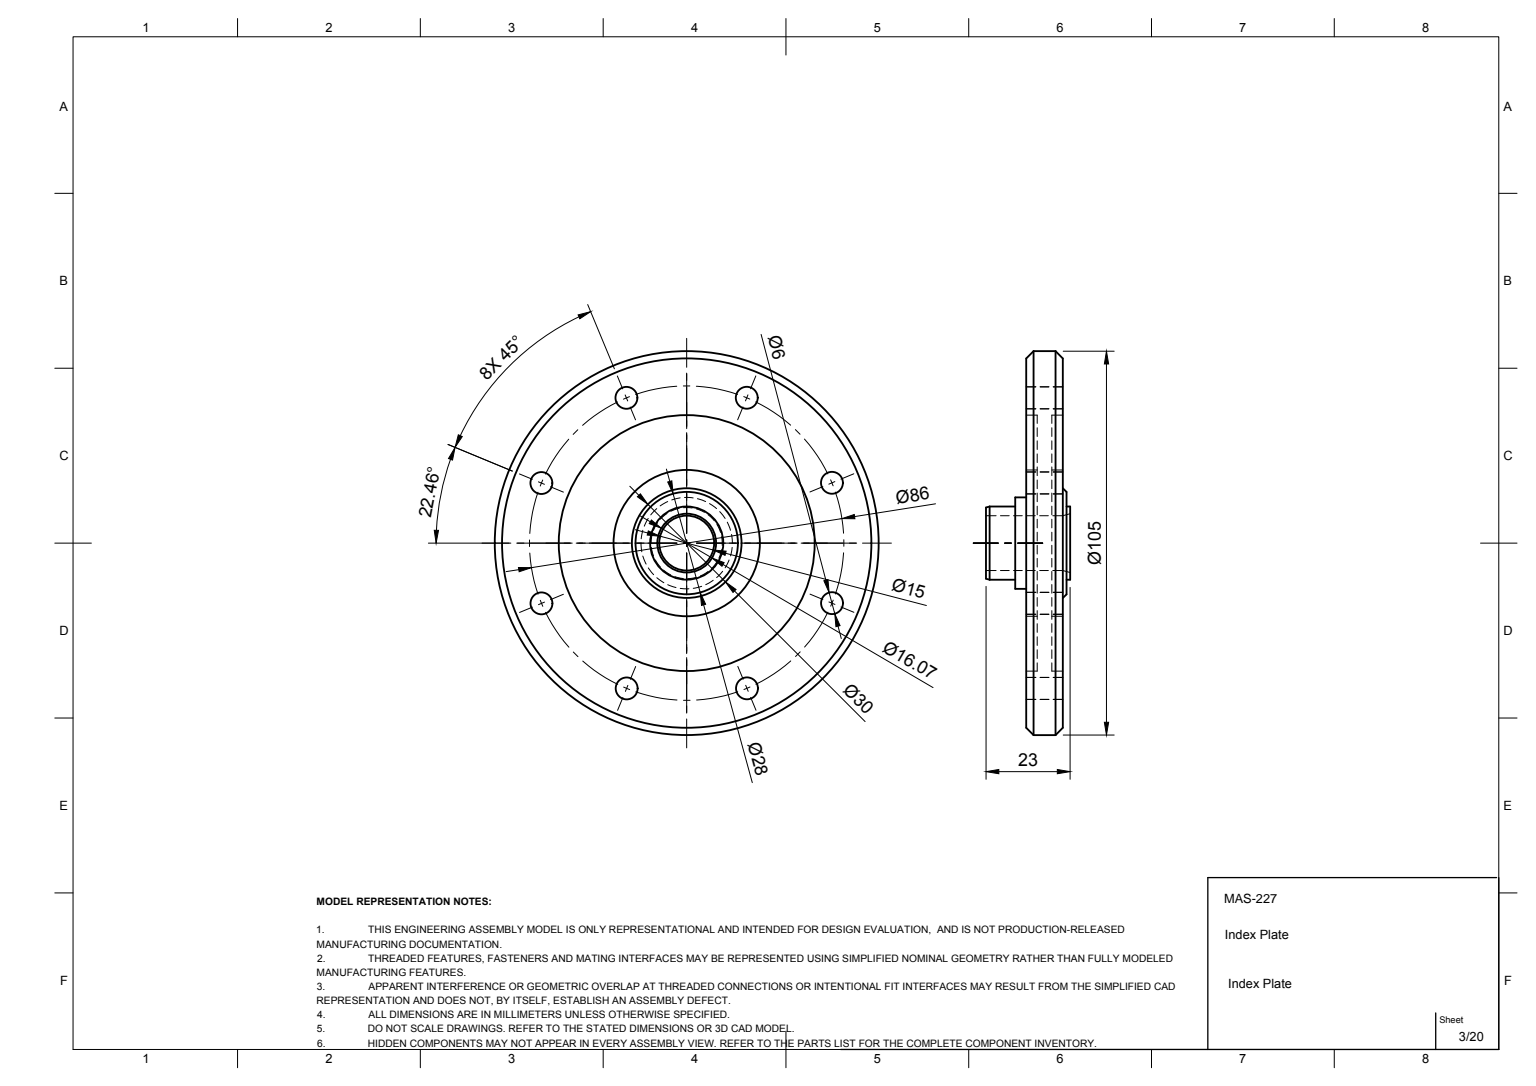
ISO-10303-21;
HEADER;
FILE_DESCRIPTION (('STEP AP214'),
    '1' );
FILE_NAME ( 'Index Plate.step', '2026-10-06T08:24:41', ( '' ), ( '' ), 'STEP AP214', 'Unspecified', '' );
FILE_SCHEMA (( 'AUTOMOTIVE_DESIGN' ));
ENDSEC;
DATA;
#10=DIRECTION ( 'NONE',  ( 0.000000000000000000, 0.000000000000000000, -1.000000000000000000 ) ) ;
#33=EDGE_CURVE ( 'NONE', #1582, #19320, #13242, .T. ) ;
#44=DIRECTION ( 'NONE',  ( -0.000000000000000000, -1.000000000000000000, -0.000000000000000000 ) ) ;
#78=VECTOR ( 'NONE', #27167, 39.37007874015748854 ) ;
#114=EDGE_CURVE ( 'NONE', #14474, #3555, #20012, .T. ) ;
#152=VERTEX_POINT ( 'NONE', #7235 ) ;
#164=CIRCLE ( 'NONE', #26696, 1.988188976448617584 ) ;
#176=ADVANCED_FACE ( 'NONE', ( #13590 ), #15218, .F. ) ;
#177=DIRECTION ( 'NONE',  ( 0.000000000000000000, 0.000000000000000000, 1.000000000000000000 ) ) ;
#193=CIRCLE ( 'NONE', #14146, 0.1181102362204720091 ) ;
#200=DIRECTION ( 'NONE',  ( 0.000000000000000000, -1.000000000000000000, 0.000000000000000000 ) ) ;
#201=DIRECTION ( 'NONE',  ( -0.000000000000000000, -1.000000000000000000, -0.000000000000000000 ) ) ;
#202=DIRECTION ( 'NONE',  ( 0.000000000000000000, 0.000000000000000000, 1.000000000000000000 ) ) ;
#247=VERTEX_POINT ( 'NONE', #23212 ) ;
#249=ORIENTED_EDGE ( 'NONE', *, *, #1427, .F. ) ;
#264=DIRECTION ( 'NONE',  ( -0.000000000000000000, -1.000000000000000000, -0.000000000000000000 ) ) ;
#291=ORIENTED_EDGE ( 'NONE', *, *, #20836, .F. ) ;
#298=EDGE_CURVE ( 'NONE', #7459, #10848, #1546, .T. ) ;
#311=ORIENTED_EDGE ( 'NONE', *, *, #16319, .F. ) ;
#320=ORIENTED_EDGE ( 'NONE', *, *, #13672, .F. ) ;
#353=DIRECTION ( 'NONE',  ( -0.000000000000000000, 1.000000000000000000, -0.000000000000000000 ) ) ;
#372=VERTEX_POINT ( 'NONE', #12604 ) ;
#378=CARTESIAN_POINT ( 'NONE',  ( 0.000000000000000000, 0.07874015746264864668, 0.000000000000000000 ) ) ;
#384=SURFACE_SIDE_STYLE ('',( #2200 ) ) ;
#403=CARTESIAN_POINT ( 'NONE',  ( 0.000000000000000000, 0.3543307086614173040, 0.000000000000000000 ) ) ;
#406=ORIENTED_EDGE ( 'NONE', *, *, #12519, .T. ) ;
#415=CARTESIAN_POINT ( 'NONE',  ( 0.000000000000000000, 0.1574803148899641958, 0.000000000000000000 ) ) ;
#436=CARTESIAN_POINT ( 'NONE',  ( 0.000000000000000000, 0.4724409448818898127, 0.000000000000000000 ) ) ;
#464=ADVANCED_FACE ( 'NONE', ( #6671 ), #22286, .T. ) ;
#482=CARTESIAN_POINT ( 'NONE',  ( 1.197070535079588716, 0.4724409448818898127, -1.315180771300060503 ) ) ;
#493=EDGE_LOOP ( 'NONE', ( #11745, #14981, #2623, #22261 ) ) ;
#508=AXIS2_PLACEMENT_3D ( 'NONE', #15619, #21831, #3001 ) ;
#514=CARTESIAN_POINT ( 'NONE',  ( 7.232166136913317628E-17, 0.07874015746264864668, -0.5905511811200284678 ) ) ;
#529=AXIS2_PLACEMENT_3D ( 'NONE', #1743, #21245, #23088 ) ;
#629=ORIENTED_EDGE ( 'NONE', *, *, #18848, .T. ) ;
#694=DIRECTION ( 'NONE',  ( -0.000000000000000000, -1.000000000000000000, -0.000000000000000000 ) ) ;
#697=ORIENTED_EDGE ( 'NONE', *, *, #23351, .F. ) ;
#706=DIRECTION ( 'NONE',  ( -0.000000000000000000, -1.000000000000000000, -0.000000000000000000 ) ) ;
#709=EDGE_CURVE ( 'NONE', #4045, #152, #22753, .T. ) ;
#726=DIRECTION ( 'NONE',  ( 0.000000000000000000, 0.000000000000000000, -1.000000000000000000 ) ) ;
#755=DIRECTION ( 'NONE',  ( -0.000000000000000000, -1.000000000000000000, -0.000000000000000000 ) ) ;
#759=PLANE ( 'NONE',  #24631 ) ;
#789=ORIENTED_EDGE ( 'NONE', *, *, #20752, .F. ) ;
#799=ORIENTED_EDGE ( 'NONE', *, *, #16948, .T. ) ;
#837=CYLINDRICAL_SURFACE ( 'NONE', #12003, 0.1181102362204718703 ) ;
#847=CARTESIAN_POINT ( 'NONE',  ( -2.073220866141732523E-16, 0.4724409448818898127, 1.692913385826771533 ) ) ;
#857=UNCERTAINTY_MEASURE_WITH_UNIT (LENGTH_MEASURE( 1.000000000000000082E-05 ), #18780, 'distance_accuracy_value', 'NONE') ;
#865=CIRCLE ( 'NONE', #10326, 0.1181102362204720091 ) ;
#870=ORIENTED_EDGE ( 'NONE', *, *, #1826, .T. ) ;
#892=DIRECTION ( 'NONE',  ( 0.000000000000000000, -1.000000000000000000, 0.000000000000000000 ) ) ;
#894=CIRCLE ( 'NONE', #26579, 0.1181102362204718703 ) ;
#911=EDGE_LOOP ( 'NONE', ( #11469, #21986 ) ) ;
#938=EDGE_LOOP ( 'NONE', ( #21430, #4636, #799, #17993 ) ) ;
#965=DIRECTION ( 'NONE',  ( 0.000000000000000000, 0.000000000000000000, -1.000000000000000000 ) ) ;
#978=AXIS2_PLACEMENT_3D ( 'NONE', #24637, #18270, #11515 ) ;
#1000=DIRECTION ( 'NONE',  ( 0.000000000000000000, -1.000000000000000000, 0.000000000000000000 ) ) ;
#1003=CARTESIAN_POINT ( 'NONE',  ( 0.000000000000000000, 0.4724409448818898127, 0.000000000000000000 ) ) ;
#1012=CARTESIAN_POINT ( 'NONE',  ( 1.197070535079588716, 0.4724409448818898127, 1.197070535079588716 ) ) ;
#1027=AXIS2_PLACEMENT_3D ( 'NONE', #3554, #3412, #20244 ) ;
#1082=CIRCLE ( 'NONE', #11898, 0.1181102362204720091 ) ;
#1086=VERTEX_POINT ( 'NONE', #20162 ) ;
#1089=ORIENTED_EDGE ( 'NONE', *, *, #4333, .F. ) ;
#1107=CARTESIAN_POINT ( 'NONE',  ( -2.073220866141732523E-16, 0.07874015748031495954, 1.574803149606299524 ) ) ;
#1178=CARTESIAN_POINT ( 'NONE',  ( 0.000000000000000000, 0.03937007874015751446, 0.5511811023975373702 ) ) ;
#1184=ORIENTED_EDGE ( 'NONE', *, *, #12547, .T. ) ;
#1222=CARTESIAN_POINT ( 'NONE',  ( 0.000000000000000000, 0.4724409448818898127, 1.377952755905512472 ) ) ;
#1244=FACE_OUTER_BOUND ( 'NONE', #1397, .T. ) ;
#1249=EDGE_CURVE ( 'NONE', #21158, #7057, #2465, .T. ) ;
#1250=EDGE_LOOP ( 'NONE', ( #8180, #21295, #4670, #1522 ) ) ;
#1298=DIRECTION ( 'NONE',  ( 0.000000000000000000, 0.000000000000000000, -1.000000000000000000 ) ) ;
#1310=AXIS2_PLACEMENT_3D ( 'NONE', #22025, #2927, #13675 ) ;
#1323=DIRECTION ( 'NONE',  ( 0.000000000000000000, -1.000000000000000000, 0.000000000000000000 ) ) ;
#1331=LINE ( 'NONE', #14195, #11270 ) ;
#1353=CIRCLE ( 'NONE', #24413, 0.1181102362204718703 ) ;
#1389=AXIS2_PLACEMENT_3D ( 'NONE', #415, #8594, #17214 ) ;
#1396=ADVANCED_FACE ( 'NONE', ( #19306 ), #27299, .F. ) ;
#1397=EDGE_LOOP ( 'NONE', ( #19459, #25159, #1953, #13540 ) ) ;
#1405=DIRECTION ( 'NONE',  ( 0.000000000000000000, 0.000000000000000000, -1.000000000000000000 ) ) ;
#1406=FACE_OUTER_BOUND ( 'NONE', #22178, .T. ) ;
#1427=EDGE_CURVE ( 'NONE', #13858, #1638, #10407, .T. ) ;
#1432=ORIENTED_EDGE ( 'NONE', *, *, #27506, .F. ) ;
#1439=FACE_OUTER_BOUND ( 'NONE', #16521, .T. ) ;
#1469=DIRECTION ( 'NONE',  ( 0.000000000000000000, 0.000000000000000000, 1.000000000000000000 ) ) ;
#1498=VERTEX_POINT ( 'NONE', #23836 ) ;
#1522=ORIENTED_EDGE ( 'NONE', *, *, #5885, .F. ) ;
#1546=CIRCLE ( 'NONE', #3787, 2.066929133858267598 ) ;
#1552=CYLINDRICAL_SURFACE ( 'NONE', #2874, 0.4921259842519685179 ) ;
#1553=CIRCLE ( 'NONE', #15987, 0.1181102362204718703 ) ;
#1582=VERTEX_POINT ( 'NONE', #514 ) ;
#1595=EDGE_LOOP ( 'NONE', ( #26419, #5301, #7926, #27061 ) ) ;
#1610=CARTESIAN_POINT ( 'NONE',  ( 1.197070535079588716, 0.4724409448818898127, -1.078960298859116707 ) ) ;
#1616=CIRCLE ( 'NONE', #19678, 0.5905511811200284678 ) ;
#1635=VECTOR ( 'NONE', #4381, 39.37007874015748143 ) ;
#1636=ORIENTED_EDGE ( 'NONE', *, *, #27592, .T. ) ;
#1638=VERTEX_POINT ( 'NONE', #14061 ) ;
#1662=ORIENTED_EDGE ( 'NONE', *, *, #10822, .F. ) ;
#1672=FACE_BOUND ( 'NONE', #15271, .T. ) ;
#1726=ADVANCED_FACE ( 'NONE', ( #26317 ), #15603, .F. ) ;
#1743=CARTESIAN_POINT ( 'NONE',  ( 1.197070535079588716, 0.07874015748031491790, 1.197070535079588716 ) ) ;
#1776=EDGE_LOOP ( 'NONE', ( #5191, #3229 ) ) ;
#1790=ORIENTED_EDGE ( 'NONE', *, *, #19478, .T. ) ;
#1813=FACE_BOUND ( 'NONE', #23770, .T. ) ;
#1820=CYLINDRICAL_SURFACE ( 'NONE', #15991, 0.1181102362204718703 ) ;
#1824=ORIENTED_EDGE ( 'NONE', *, *, #3257, .F. ) ;
#1826=EDGE_CURVE ( 'NONE', #17190, #19458, #11615, .T. ) ;
#1845=DIRECTION ( 'NONE',  ( 0.000000000000000000, -1.000000000000000000, 0.000000000000000000 ) ) ;
#1864=CIRCLE ( 'NONE', #3209, 0.1181102362204718703 ) ;
#1930=AXIS2_PLACEMENT_3D ( 'NONE', #8276, #16896, #4038 ) ;
#1938=EDGE_LOOP ( 'NONE', ( #18405, #23530, #16825, #17076 ) ) ;
#1939=AXIS2_PLACEMENT_3D ( 'NONE', #16280, #5401, #14020 ) ;
#1953=ORIENTED_EDGE ( 'NONE', *, *, #18523, .F. ) ;
#1991=ORIENTED_EDGE ( 'NONE', *, *, #20752, .T. ) ;
#2060=VECTOR ( 'NONE', #15684, 39.37007874015748143 ) ;
#2102=CARTESIAN_POINT ( 'NONE',  ( 0.000000000000000000, 0.9055118110236221041, 0.000000000000000000 ) ) ;
#2122=ORIENTED_EDGE ( 'NONE', *, *, #5680, .F. ) ;
#2124=AXIS2_PLACEMENT_3D ( 'NONE', #13217, #12672, #11106 ) ;
#2135=ORIENTED_EDGE ( 'NONE', *, *, #21289, .T. ) ;
#2145=( GEOMETRIC_REPRESENTATION_CONTEXT ( 3 ) GLOBAL_UNCERTAINTY_ASSIGNED_CONTEXT ( ( #24851 ) ) GLOBAL_UNIT_ASSIGNED_CONTEXT ( ( #26069, #23822, #10819 ) ) REPRESENTATION_CONTEXT ( 'NONE', 'WORKASPACE' ) ) ;
#2170=CARTESIAN_POINT ( 'NONE',  ( 0.000000000000000000, 0.07874015748662489822, 0.000000000000000000 ) ) ;
#2181=EDGE_LOOP ( 'NONE', ( #2379, #22153 ) ) ;
#2186=LINE ( 'NONE', #14929, #19182 ) ;
#2194=LINE ( 'NONE', #8827, #18525 ) ;
#2200=SURFACE_STYLE_FILL_AREA ( #4325 ) ;
#2225=VERTEX_POINT ( 'NONE', #20456 ) ;
#2314=FACE_OUTER_BOUND ( 'NONE', #19001, .T. ) ;
#2328=( LENGTH_UNIT ( ) NAMED_UNIT ( * ) SI_UNIT ( $, .METRE. ) ) ;
#2332=CYLINDRICAL_SURFACE ( 'NONE', #25371, 0.1181102362204718703 ) ;
#2379=ORIENTED_EDGE ( 'NONE', *, *, #15595, .T. ) ;
#2409=AXIS2_PLACEMENT_3D ( 'NONE', #403, #13231, #17610 ) ;
#2460=DIRECTION ( 'NONE',  ( 0.000000000000000000, 0.000000000000000000, -1.000000000000000000 ) ) ;
#2465=CIRCLE ( 'NONE', #2913, 1.988188976307287970 ) ;
#2480=ORIENTED_EDGE ( 'NONE', *, *, #12460, .F. ) ;
#2514=CIRCLE ( 'NONE', #22359, 0.1181102362204718703 ) ;
#2527=DIRECTION ( 'NONE',  ( 0.000000000000000000, 0.000000000000000000, -1.000000000000000000 ) ) ;
#2543=CARTESIAN_POINT ( 'NONE',  ( 1.692913385826771533, 0.4724409448818898127, 0.1181102362204723144 ) ) ;
#2550=EDGE_LOOP ( 'NONE', ( #23716, #23135, #18608, #25264 ) ) ;
#2576=APPLICATION_CONTEXT ( 'automotive_design' ) ;
#2623=ORIENTED_EDGE ( 'NONE', *, *, #25477, .T. ) ;
#2674=ADVANCED_FACE ( 'NONE', ( #8431 ), #10402, .T. ) ;
#2689=ORIENTED_EDGE ( 'NONE', *, *, #22485, .T. ) ;
#2707=MANIFOLD_SOLID_BREP ( 'Index Plate', #6943 ) ;
#2718=ORIENTED_EDGE ( 'NONE', *, *, #10592, .T. ) ;
#2741=CIRCLE ( 'NONE', #978, 0.3831516066089791228 ) ;
#2769=FACE_OUTER_BOUND ( 'NONE', #11806, .T. ) ;
#2772=CONICAL_SURFACE ( 'NONE', #11805, 1.988188976307287970, 0.7853981642948970610 ) ;
#2776=DIRECTION ( 'NONE',  ( -0.000000000000000000, 1.000000000000000000, -0.000000000000000000 ) ) ;
#2782=LINE ( 'NONE', #11011, #8118 ) ;
#2784=EDGE_CURVE ( 'NONE', #13707, #10268, #25934, .T. ) ;
#2794=CIRCLE ( 'NONE', #3231, 0.7874015748031496509 ) ;
#2796=CARTESIAN_POINT ( 'NONE',  ( 0.000000000000000000, 0.1968503937007874127, -0.3937007874015748254 ) ) ;
#2812=EDGE_CURVE ( 'NONE', #2225, #7703, #23380, .T. ) ;
#2835=CARTESIAN_POINT ( 'NONE',  ( 0.000000000000000000, 0.07874015746264864668, 0.5905511811200284678 ) ) ;
#2845=LINE ( 'NONE', #11483, #16951 ) ;
#2851=DIRECTION ( 'NONE',  ( 0.000000000000000000, 0.000000000000000000, -1.000000000000000000 ) ) ;
#2874=AXIS2_PLACEMENT_3D ( 'NONE', #10156, #27408, #8066 ) ;
#2875=ORIENTED_EDGE ( 'NONE', *, *, #4475, .T. ) ;
#2878=AXIS2_PLACEMENT_3D ( 'NONE', #378, #3646, #18474 ) ;
#2898=ORIENTED_EDGE ( 'NONE', *, *, #24019, .F. ) ;
#2913=AXIS2_PLACEMENT_3D ( 'NONE', #14096, #26953, #965 ) ;
#2927=DIRECTION ( 'NONE',  ( -0.000000000000000000, -1.000000000000000000, -0.000000000000000000 ) ) ;
#2933=DIMENSIONAL_EXPONENTS ( 1.000000000000000000, 0.000000000000000000, 0.000000000000000000, 0.000000000000000000, 0.000000000000000000, 0.000000000000000000, 0.000000000000000000 ) ;
#2961=EDGE_LOOP ( 'NONE', ( #5163, #7139, #19666, #17295 ) ) ;
#2970=EDGE_LOOP ( 'NONE', ( #22132, #13262 ) ) ;
#2973=EDGE_CURVE ( 'NONE', #18986, #1498, #26337, .T. ) ;
#3000=DIRECTION ( 'NONE',  ( -0.000000000000000000, -1.000000000000000000, -0.000000000000000000 ) ) ;
#3001=DIRECTION ( 'NONE',  ( 0.000000000000000000, 0.000000000000000000, -1.000000000000000000 ) ) ;
#3013=STYLED_ITEM ( 'NONE', ( #6589 ), #2707 ) ;
#3036=AXIS2_PLACEMENT_3D ( 'NONE', #19500, #25728, #6375 ) ;
#3043=DIRECTION ( 'NONE',  ( -0.000000000000000000, -1.000000000000000000, -0.000000000000000000 ) ) ;
#3055=AXIS2_PLACEMENT_3D ( 'NONE', #14460, #3688, #12316 ) ;
#3068=EDGE_LOOP ( 'NONE', ( #12674, #2875, #25773, #20146 ) ) ;
#3069=ADVANCED_FACE ( 'NONE', ( #6279 ), #14838, .F. ) ;
#3070=ORIENTED_EDGE ( 'NONE', *, *, #9051, .T. ) ;
#3095=LENGTH_MEASURE_WITH_UNIT ( LENGTH_MEASURE( 0.02539999999999999897 ), #22747 ) ;
#3120=EDGE_CURVE ( 'NONE', #7099, #13627, #22918, .T. ) ;
#3122=AXIS2_PLACEMENT_3D ( 'NONE', #20332, #24693, #13985 ) ;
#3168=DIRECTION ( 'NONE',  ( 0.000000000000000000, -1.000000000000000000, 0.000000000000000000 ) ) ;
#3201=VERTEX_POINT ( 'NONE', #18103 ) ;
#3209=AXIS2_PLACEMENT_3D ( 'NONE', #3734, #14648, #3882 ) ;
#3216=CARTESIAN_POINT ( 'NONE',  ( 0.000000000000000000, 0.5905511811023621549, 0.000000000000000000 ) ) ;
#3223=CARTESIAN_POINT ( 'NONE',  ( -1.197070535079588716, 0.4724409448818898127, -1.078960298859116707 ) ) ;
#3224=FACE_OUTER_BOUND ( 'NONE', #18819, .T. ) ;
#3229=ORIENTED_EDGE ( 'NONE', *, *, #19328, .T. ) ;
#3231=AXIS2_PLACEMENT_3D ( 'NONE', #10033, #1845, #10310 ) ;
#3244=ADVANCED_FACE ( 'NONE', ( #18257 ), #7258, .F. ) ;
#3245=DIRECTION ( 'NONE',  ( 0.000000000000000000, 0.000000000000000000, -1.000000000000000000 ) ) ;
#3257=EDGE_CURVE ( 'NONE', #372, #13858, #19762, .T. ) ;
#3379=VECTOR ( 'NONE', #4006, 39.37007874015748854 ) ;
#3403=DIRECTION ( 'NONE',  ( -0.000000000000000000, -1.000000000000000000, -0.000000000000000000 ) ) ;
#3412=DIRECTION ( 'NONE',  ( -0.000000000000000000, 1.000000000000000000, -0.000000000000000000 ) ) ;
#3415=EDGE_LOOP ( 'NONE', ( #27420, #16968 ) ) ;
#3459=EDGE_LOOP ( 'NONE', ( #14828, #18126 ) ) ;
#3471=CARTESIAN_POINT ( 'NONE',  ( 1.446433227339386678E-17, 0.4724409448818898127, -1.574803149606299524 ) ) ;
#3477=ORIENTED_EDGE ( 'NONE', *, *, #8160, .T. ) ;
#3478=DIRECTION ( 'NONE',  ( 0.000000000000000000, -1.000000000000000000, 0.000000000000000000 ) ) ;
#3479=DIRECTION ( 'NONE',  ( -0.000000000000000000, -1.000000000000000000, -0.000000000000000000 ) ) ;
#3480=DIRECTION ( 'NONE',  ( 0.000000000000000000, -0.9659258263664941557, -0.2588190448135637145 ) ) ;
#3494=EDGE_CURVE ( 'NONE', #23576, #24515, #4893, .T. ) ;
#3513=DIRECTION ( 'NONE',  ( -0.000000000000000000, -1.000000000000000000, -0.000000000000000000 ) ) ;
#3525=DIRECTION ( 'NONE',  ( -0.000000000000000000, -1.000000000000000000, -0.000000000000000000 ) ) ;
#3530=AXIS2_PLACEMENT_3D ( 'NONE', #9173, #7487, #22603 ) ;
#3544=LINE ( 'NONE', #5262, #78 ) ;
#3551=VECTOR ( 'NONE', #16165, 39.37007874015748143 ) ;
#3554=CARTESIAN_POINT ( 'NONE',  ( 0.000000000000000000, 0.4724409448818896462, 0.000000000000000000 ) ) ;
#3555=VERTEX_POINT ( 'NONE', #1610 ) ;
#3606=ADVANCED_BREP_SHAPE_REPRESENTATION ( 'Index Plate', ( #2707, #11588 ), #8455 ) ;
#3618=CIRCLE ( 'NONE', #21691, 0.3937007874015748254 ) ;
#3638=ORIENTED_EDGE ( 'NONE', *, *, #20353, .F. ) ;
#3646=DIRECTION ( 'NONE',  ( 0.000000000000000000, -1.000000000000000000, 0.000000000000000000 ) ) ;
#3665=DIRECTION ( 'NONE',  ( 0.000000000000000000, 0.000000000000000000, 1.000000000000000000 ) ) ;
#3672=CARTESIAN_POINT ( 'NONE',  ( -1.692913385826771533, 0.07874015748031491790, 0.1181102362204718981 ) ) ;
#3680=CYLINDRICAL_SURFACE ( 'NONE', #9596, 0.1181102362204718703 ) ;
#3685=EDGE_CURVE ( 'NONE', #16564, #8713, #6703, .T. ) ;
#3688=DIRECTION ( 'NONE',  ( 0.000000000000000000, -1.000000000000000000, 0.000000000000000000 ) ) ;
#3695=CIRCLE ( 'NONE', #2409, 0.7874015748031496509 ) ;
#3716=FACE_OUTER_BOUND ( 'NONE', #16941, .T. ) ;
#3734=CARTESIAN_POINT ( 'NONE',  ( -1.197070535079588716, 0.07874015748031491790, -1.197070535079588716 ) ) ;
#3736=ORIENTED_EDGE ( 'NONE', *, *, #298, .F. ) ;
#3749=CARTESIAN_POINT ( 'NONE',  ( 0.000000000000000000, 0.5905511811023621549, 0.000000000000000000 ) ) ;
#3762=CARTESIAN_POINT ( 'NONE',  ( 0.000000000000000000, 0.3543307086614172485, 1.377952755905512472 ) ) ;
#3787=AXIS2_PLACEMENT_3D ( 'NONE', #6123, #7950, #14758 ) ;
#3794=ORIENTED_EDGE ( 'NONE', *, *, #11136, .F. ) ;
#3815=CARTESIAN_POINT ( 'NONE',  ( 4.756848988674917118E-17, 0.9055118110236221041, 0.3831516066089791228 ) ) ;
#3846=VECTOR ( 'NONE', #3403, 39.37007874015748143 ) ;
#3856=CARTESIAN_POINT ( 'NONE',  ( 0.000000000000000000, 0.07874015748662489822, 0.000000000000000000 ) ) ;
#3866=DIRECTION ( 'NONE',  ( 0.000000000000000000, -1.000000000000000000, 0.000000000000000000 ) ) ;
#3882=DIRECTION ( 'NONE',  ( 0.000000000000000000, 0.000000000000000000, -1.000000000000000000 ) ) ;
#3899=CARTESIAN_POINT ( 'NONE',  ( 0.000000000000000000, 0.07874015748031491790, -1.692913385826771533 ) ) ;
#3906=FACE_OUTER_BOUND ( 'NONE', #14752, .T. ) ;
#3934=VERTEX_POINT ( 'NONE', #19157 ) ;
#3937=DIRECTION ( 'NONE',  ( -0.000000000000000000, 1.000000000000000000, -0.000000000000000000 ) ) ;
#3946=ORIENTED_EDGE ( 'NONE', *, *, #16858, .F. ) ;
#3956=DIRECTION ( 'NONE',  ( 0.000000000000000000, 0.000000000000000000, -1.000000000000000000 ) ) ;
#3960=EDGE_LOOP ( 'NONE', ( #697, #25923 ) ) ;
#3981=ORIENTED_EDGE ( 'NONE', *, *, #2973, .F. ) ;
#4006=DIRECTION ( 'NONE',  ( 0.000000000000000000, -0.9659258263664933786, -0.2588190448135661570 ) ) ;
#4038=DIRECTION ( 'NONE',  ( 0.000000000000000000, 0.000000000000000000, -1.000000000000000000 ) ) ;
#4045=VERTEX_POINT ( 'NONE', #18047 ) ;
#4048=DIRECTION ( 'NONE',  ( 0.000000000000000000, 1.000000000000000000, 0.000000000000000000 ) ) ;
#4055=FACE_OUTER_BOUND ( 'NONE', #10449, .T. ) ;
#4060=ADVANCED_FACE ( 'NONE', ( #1244 ), #7157, .T. ) ;
#4079=CARTESIAN_POINT ( 'NONE',  ( 0.000000000000000000, 0.3543307086614172485, 0.000000000000000000 ) ) ;
#4125=FACE_OUTER_BOUND ( 'NONE', #4418, .T. ) ;
#4141=ORIENTED_EDGE ( 'NONE', *, *, #22416, .F. ) ;
#4161=CIRCLE ( 'NONE', #7316, 0.3937007874015748254 ) ;
#4228=FACE_OUTER_BOUND ( 'NONE', #1938, .T. ) ;
#4269=AXIS2_PLACEMENT_3D ( 'NONE', #3856, #1323, #16998 ) ;
#4325=FILL_AREA_STYLE ('',( #23421 ) ) ;
#4333=EDGE_CURVE ( 'NONE', #27329, #8591, #12247, .T. ) ;
#4366=CIRCLE ( 'NONE', #14290, 0.3937007874015748254 ) ;
#4381=DIRECTION ( 'NONE',  ( 0.000000000000000000, -1.000000000000000000, 0.000000000000000000 ) ) ;
#4405=CARTESIAN_POINT ( 'NONE',  ( 0.000000000000000000, 0.4724409448818898127, -1.692913385826771533 ) ) ;
#4418=EDGE_LOOP ( 'NONE', ( #6913, #20985, #27516, #4926 ) ) ;
#4435=FACE_OUTER_BOUND ( 'NONE', #1595, .T. ) ;
#4437=DIRECTION ( 'NONE',  ( 0.000000000000000000, -1.000000000000000000, 0.000000000000000000 ) ) ;
#4454=CARTESIAN_POINT ( 'NONE',  ( 0.000000000000000000, 0.07874015748031495954, 0.000000000000000000 ) ) ;
#4457=CARTESIAN_POINT ( 'NONE',  ( 0.000000000000000000, 0.1968503937007875237, 0.000000000000000000 ) ) ;
#4459=AXIS2_PLACEMENT_3D ( 'NONE', #23177, #16518, #18915 ) ;
#4469=ORIENTED_EDGE ( 'NONE', *, *, #3494, .F. ) ;
#4471=ADVANCED_FACE ( 'NONE', ( #4435 ), #21112, .T. ) ;
#4475=EDGE_CURVE ( 'NONE', #14551, #1582, #13040, .T. ) ;
#4504=AXIS2_PLACEMENT_3D ( 'NONE', #21973, #13349, #4725 ) ;
#4547=AXIS2_PLACEMENT_3D ( 'NONE', #5748, #14365, #23119 ) ;
#4556=AXIS2_PLACEMENT_3D ( 'NONE', #4457, #4048, #10531 ) ;
#4560=CARTESIAN_POINT ( 'NONE',  ( 0.000000000000000000, 0.4724409448818898127, 0.000000000000000000 ) ) ;
#4588=DIRECTION ( 'NONE',  ( -0.000000000000000000, 1.000000000000000000, -0.000000000000000000 ) ) ;
#4612=SHAPE_REPRESENTATION ( 'Index Plate', ( #11588 ), #8455 ) ;
#4615=ORIENTED_EDGE ( 'NONE', *, *, #5314, .T. ) ;
#4636=ORIENTED_EDGE ( 'NONE', *, *, #16319, .T. ) ;
#4670=ORIENTED_EDGE ( 'NONE', *, *, #25230, .T. ) ;
#4676=PLANE ( 'NONE',  #18658 ) ;
#4713=ADVANCED_FACE ( 'NONE', ( #21219 ), #23418, .T. ) ;
#4714=DIRECTION ( 'NONE',  ( 0.000000000000000000, 0.000000000000000000, -1.000000000000000000 ) ) ;
#4718=FACE_OUTER_BOUND ( 'NONE', #9689, .T. ) ;
#4725=DIRECTION ( 'NONE',  ( 0.000000000000000000, 0.000000000000000000, 1.000000000000000000 ) ) ;
#4726=ADVANCED_FACE ( 'NONE', ( #4125 ), #13008, .F. ) ;
#4757=CARTESIAN_POINT ( 'NONE',  ( 9.642888182262624280E-17, 0.4724409448818898127, 0.7874015748031496509 ) ) ;
#4759=CARTESIAN_POINT ( 'NONE',  ( 0.7874015748031496509, 0.4724409448818898127, 0.000000000000000000 ) ) ;
#4789=DIRECTION ( 'NONE',  ( -0.000000000000000000, -1.000000000000000000, -0.000000000000000000 ) ) ;
#4801=DIRECTION ( 'NONE',  ( 0.000000000000000000, -1.000000000000000000, 0.000000000000000000 ) ) ;
#4812=CIRCLE ( 'NONE', #22864, 0.3937007874015748254 ) ;
#4838=CARTESIAN_POINT ( 'NONE',  ( 0.000000000000000000, 0.07874015748031495954, 0.000000000000000000 ) ) ;
#4876=EDGE_CURVE ( 'NONE', #17502, #8729, #24952, .T. ) ;
#4880=EDGE_LOOP ( 'NONE', ( #7922, #25227 ) ) ;
#4893=CIRCLE ( 'NONE', #22482, 0.1181102362204720091 ) ;
#4926=ORIENTED_EDGE ( 'NONE', *, *, #25976, .F. ) ;
#4931=AXIS2_PLACEMENT_3D ( 'NONE', #23558, #17182, #23423 ) ;
#4933=DIRECTION ( 'NONE',  ( 0.000000000000000000, -1.000000000000000000, 0.000000000000000000 ) ) ;
#4939=FACE_BOUND ( 'NONE', #27144, .T. ) ;
#4974=AXIS2_PLACEMENT_3D ( 'NONE', #9963, #6026, #18565 ) ;
#4978=CARTESIAN_POINT ( 'NONE',  ( 1.197070535079588716, 0.07874015748031491790, -1.315180771300060503 ) ) ;
#4983=EDGE_CURVE ( 'NONE', #10848, #1086, #11751, .T. ) ;
#4994=CYLINDRICAL_SURFACE ( 'NONE', #12683, 0.1181102362204718703 ) ;
#5025=CIRCLE ( 'NONE', #19920, 1.377952755905512472 ) ;
#5079=PRODUCT_DEFINITION_SHAPE ( 'NONE', 'NONE',  #6545 ) ;
#5082=AXIS2_PLACEMENT_3D ( 'NONE', #5721, #25337, #1469 ) ;
#5091=DIRECTION ( 'NONE',  ( 0.000000000000000000, 0.000000000000000000, 1.000000000000000000 ) ) ;
#5092=ORIENTED_EDGE ( 'NONE', *, *, #10873, .T. ) ;
#5116=DIRECTION ( 'NONE',  ( -0.000000000000000000, 1.000000000000000000, -0.000000000000000000 ) ) ;
#5154=ADVANCED_FACE ( 'NONE', ( #1439 ), #7948, .T. ) ;
#5163=ORIENTED_EDGE ( 'NONE', *, *, #23351, .T. ) ;
#5171=AXIS2_PLACEMENT_3D ( 'NONE', #27510, #18866, #6184 ) ;
#5191=ORIENTED_EDGE ( 'NONE', *, *, #1249, .T. ) ;
#5192=EDGE_CURVE ( 'NONE', #27168, #3201, #14400, .T. ) ;
#5220=ADVANCED_FACE ( 'NONE', ( #3224, #26412 ), #22182, .T. ) ;
#5221=AXIS2_PLACEMENT_3D ( 'NONE', #25419, #6219, #6393 ) ;
#5229=CARTESIAN_POINT ( 'NONE',  ( 0.000000000000000000, 0.000000000000000000, 0.000000000000000000 ) ) ;
#5232=FACE_OUTER_BOUND ( 'NONE', #16959, .T. ) ;
#5236=LINE ( 'NONE', #16266, #25041 ) ;
#5252=EDGE_CURVE ( 'NONE', #8729, #15321, #27474, .T. ) ;
#5257=CARTESIAN_POINT ( 'NONE',  ( 1.197070535079588716, 0.4724409448818898127, -1.197070535079588716 ) ) ;
#5262=CARTESIAN_POINT ( 'NONE',  ( 2.531258147843938596E-16, 0.3937007873309092409, 2.066929133858267598 ) ) ;
#5292=ORIENTED_EDGE ( 'NONE', *, *, #19478, .F. ) ;
#5301=ORIENTED_EDGE ( 'NONE', *, *, #1249, .F. ) ;
#5307=ORIENTED_EDGE ( 'NONE', *, *, #15668, .T. ) ;
#5314=EDGE_CURVE ( 'NONE', #21174, #27329, #26114, .T. ) ;
#5326=DIRECTION ( 'NONE',  ( 0.000000000000000000, -1.000000000000000000, 0.000000000000000000 ) ) ;
#5328=DIRECTION ( 'NONE',  ( -0.000000000000000000, -1.000000000000000000, -0.000000000000000000 ) ) ;
#5376=FACE_OUTER_BOUND ( 'NONE', #5601, .T. ) ;
#5377=DIRECTION ( 'NONE',  ( -0.000000000000000000, 1.000000000000000000, -0.000000000000000000 ) ) ;
#5401=DIRECTION ( 'NONE',  ( -0.000000000000000000, 1.000000000000000000, -0.000000000000000000 ) ) ;
#5420=EDGE_LOOP ( 'NONE', ( #26664, #25848 ) ) ;
#5459=DIRECTION ( 'NONE',  ( 0.000000000000000000, 0.000000000000000000, -1.000000000000000000 ) ) ;
#5563=ORIENTED_EDGE ( 'NONE', *, *, #26212, .T. ) ;
#5593=CARTESIAN_POINT ( 'NONE',  ( 1.197070535079588716, 0.07874015748031491790, 1.315180771300060503 ) ) ;
#5594=LINE ( 'NONE', #1222, #6450 ) ;
#5601=EDGE_LOOP ( 'NONE', ( #11782, #25405, #3477, #10617 ) ) ;
#5620=EDGE_LOOP ( 'NONE', ( #20522, #13116, #10840, #13234 ) ) ;
#5621=LINE ( 'NONE', #21395, #16197 ) ;
#5636=VECTOR ( 'NONE', #20203, 39.37007874015748143 ) ;
#5649=EDGE_CURVE ( 'NONE', #12934, #3201, #5621, .T. ) ;
#5660=CYLINDRICAL_SURFACE ( 'NONE', #11486, 0.2952755905511805778 ) ;
#5666=EDGE_LOOP ( 'NONE', ( #4615, #16993 ) ) ;
#5669=DIRECTION ( 'NONE',  ( 0.000000000000000000, 0.000000000000000000, -1.000000000000000000 ) ) ;
#5680=EDGE_CURVE ( 'NONE', #22837, #17502, #17087, .T. ) ;
#5721=CARTESIAN_POINT ( 'NONE',  ( 0.4921259842519685179, 0.5905511811023621549, 0.000000000000000000 ) ) ;
#5729=AXIS2_PLACEMENT_3D ( 'NONE', #9022, #19640, #24147 ) ;
#5736=ORIENTED_EDGE ( 'NONE', *, *, #26852, .F. ) ;
#5741=AXIS2_PLACEMENT_3D ( 'NONE', #23293, #5377, #18201 ) ;
#5748=CARTESIAN_POINT ( 'NONE',  ( -1.197070535079588716, 0.07874015748031495954, -1.197070535079588716 ) ) ;
#5756=CARTESIAN_POINT ( 'NONE',  ( 0.000000000000000000, 0.4724409448818898127, -1.811023622047243542 ) ) ;
#5762=DIRECTION ( 'NONE',  ( 0.000000000000000000, 0.000000000000000000, -1.000000000000000000 ) ) ;
#5783=ORIENTED_EDGE ( 'NONE', *, *, #7586, .F. ) ;
#5799=DIRECTION ( 'NONE',  ( 0.000000000000000000, -0.7071067818211396183, -0.7071067805519553051 ) ) ;
#5804=AXIS2_PLACEMENT_3D ( 'NONE', #12901, #11063, #19813 ) ;
#5807=ORIENTED_EDGE ( 'NONE', *, *, #26124, .F. ) ;
#5824=FACE_OUTER_BOUND ( 'NONE', #5620, .T. ) ;
#5885=EDGE_CURVE ( 'NONE', #16430, #4045, #24633, .T. ) ;
#5926=DIRECTION ( 'NONE',  ( 0.000000000000000000, 0.000000000000000000, 1.000000000000000000 ) ) ;
#5962=AXIS2_PLACEMENT_3D ( 'NONE', #25760, #19682, #19255 ) ;
#6023=ORIENTED_EDGE ( 'NONE', *, *, #17691, .T. ) ;
#6026=DIRECTION ( 'NONE',  ( -0.000000000000000000, -1.000000000000000000, -0.000000000000000000 ) ) ;
#6049=CIRCLE ( 'NONE', #21825, 0.3937007874015748254 ) ;
#6053=CARTESIAN_POINT ( 'NONE',  ( 0.000000000000000000, 0.07874015748662489822, 0.000000000000000000 ) ) ;
#6123=CARTESIAN_POINT ( 'NONE',  ( 0.000000000000000000, 0.3937007873309092409, 0.000000000000000000 ) ) ;
#6136=DIRECTION ( 'NONE',  ( 0.000000000000000000, -1.000000000000000000, 0.000000000000000000 ) ) ;
#6145=DIRECTION ( 'NONE',  ( 0.000000000000000000, 1.000000000000000000, 0.000000000000000000 ) ) ;
#6178=FACE_OUTER_BOUND ( 'NONE', #13209, .T. ) ;
#6184=DIRECTION ( 'NONE',  ( 0.000000000000000000, 0.000000000000000000, -1.000000000000000000 ) ) ;
#6206=ORIENTED_EDGE ( 'NONE', *, *, #27465, .T. ) ;
#6219=DIRECTION ( 'NONE',  ( -0.000000000000000000, -1.000000000000000000, -0.000000000000000000 ) ) ;
#6230=EDGE_LOOP ( 'NONE', ( #8621, #24988 ) ) ;
#6279=FACE_OUTER_BOUND ( 'NONE', #9688, .T. ) ;
#6337=ORIENTED_EDGE ( 'NONE', *, *, #4876, .T. ) ;
#6342=FACE_BOUND ( 'NONE', #6230, .T. ) ;
#6344=ORIENTED_EDGE ( 'NONE', *, *, #7766, .F. ) ;
#6375=DIRECTION ( 'NONE',  ( 0.000000000000000000, 0.000000000000000000, -1.000000000000000000 ) ) ;
#6389=DIRECTION ( 'NONE',  ( 0.000000000000000000, 0.000000000000000000, -1.000000000000000000 ) ) ;
#6393=DIRECTION ( 'NONE',  ( 0.000000000000000000, 0.000000000000000000, -1.000000000000000000 ) ) ;
#6399=ADVANCED_FACE ( 'NONE', ( #19295, #25521 ), #25797, .T. ) ;
#6405=FACE_BOUND ( 'NONE', #17549, .T. ) ;
#6421=ADVANCED_FACE ( 'NONE', ( #3906 ), #14813, .F. ) ;
#6450=VECTOR ( 'NONE', #9825, 39.37007874015748143 ) ;
#6476=ORIENTED_EDGE ( 'NONE', *, *, #25477, .F. ) ;
#6531=DIRECTION ( 'NONE',  ( -0.000000000000000000, -1.000000000000000000, -0.000000000000000000 ) ) ;
#6545=PRODUCT_DEFINITION ( 'UNKNOWN', '', #14348, #23796 ) ;
#6552=ADVANCED_FACE ( 'NONE', ( #11507 ), #17126, .T. ) ;
#6589=PRESENTATION_STYLE_ASSIGNMENT (( #21553 ) ) ;
#6614=VERTEX_POINT ( 'NONE', #14388 ) ;
#6616=CIRCLE ( 'NONE', #21494, 0.7874015748208159637 ) ;
#6633=VECTOR ( 'NONE', #14478, 39.37007874015748143 ) ;
#6639=CARTESIAN_POINT ( 'NONE',  ( 1.197070535079588716, 0.4724409448818898127, -1.197070535079588716 ) ) ;
#6654=DIRECTION ( 'NONE',  ( 0.000000000000000000, -1.000000000000000000, 0.000000000000000000 ) ) ;
#6671=FACE_OUTER_BOUND ( 'NONE', #21866, .T. ) ;
#6673=CARTESIAN_POINT ( 'NONE',  ( 0.000000000000000000, 0.07874015748031491790, -1.692913385826771533 ) ) ;
#6690=ORIENTED_EDGE ( 'NONE', *, *, #8529, .T. ) ;
#6702=AXIS2_PLACEMENT_3D ( 'NONE', #27359, #27504, #16611 ) ;
#6703=CIRCLE ( 'NONE', #5804, 0.3163739521363750362 ) ;
#6709=EDGE_CURVE ( 'NONE', #8713, #16564, #12628, .T. ) ;
#6784=CYLINDRICAL_SURFACE ( 'NONE', #9269, 0.1181102362204720091 ) ;
#6796=ORIENTED_EDGE ( 'NONE', *, *, #11893, .T. ) ;
#6797=DIRECTION ( 'NONE',  ( 0.000000000000000000, -1.000000000000000000, 0.000000000000000000 ) ) ;
#6803=CIRCLE ( 'NONE', #1389, 2.066929133858267598 ) ;
#6806=DIRECTION ( 'NONE',  ( -0.000000000000000000, -1.000000000000000000, -0.000000000000000000 ) ) ;
#6835=EDGE_CURVE ( 'NONE', #17724, #26290, #13546, .T. ) ;
#6839=AXIS2_PLACEMENT_3D ( 'NONE', #13373, #11526, #15909 ) ;
#6849=CARTESIAN_POINT ( 'NONE',  ( 0.000000000000000000, 0.07874015746264864668, 0.000000000000000000 ) ) ;
#6913=ORIENTED_EDGE ( 'NONE', *, *, #13672, .T. ) ;
#6943=CLOSED_SHELL ( 'NONE', ( #464, #3069, #4060, #8477, #3244, #4726, #13143, #21782, #24844, #27055, #7859, #10937, #15660, #5154, #8461, #24780, #6552, #15723, #2674, #1726, #15050, #20764, #17607, #11427, #24289, #23830, #9727, #7669, #20923, #23178, #23527, #26593, #6399, #4713, #5220, #15053, #19864, #26550, #24917, #15310, #9513, #10160, #176, #26993, #7893, #8259, #23826, #11945, #6421, #15147, #4471, #20738, #1396, #15306 ) ) ;
#6953=DIRECTION ( 'NONE',  ( 0.000000000000000000, -1.000000000000000000, 0.000000000000000000 ) ) ;
#6995=CYLINDRICAL_SURFACE ( 'NONE', #508, 0.1181102362204720091 ) ;
#7048=DIRECTION ( 'NONE',  ( 0.000000000000000000, 0.7071067811865474617, 0.7071067811865474617 ) ) ;
#7057=VERTEX_POINT ( 'NONE', #27543 ) ;
#7066=DIRECTION ( 'NONE',  ( 0.000000000000000000, 0.000000000000000000, -1.000000000000000000 ) ) ;
#7067=DIRECTION ( 'NONE',  ( -0.000000000000000000, -1.000000000000000000, -0.000000000000000000 ) ) ;
#7099=VERTEX_POINT ( 'NONE', #4757 ) ;
#7128=CARTESIAN_POINT ( 'NONE',  ( 0.000000000000000000, 0.07874015748031491790, -1.811023622047243542 ) ) ;
#7139=ORIENTED_EDGE ( 'NONE', *, *, #15537, .T. ) ;
#7157=CONICAL_SURFACE ( 'NONE', #7629, 2.066929133858267598, 0.7853981624999996081 ) ;
#7165=VECTOR ( 'NONE', #18715, 39.37007874015748143 ) ;
#7166=PLANE ( 'NONE',  #26346 ) ;
#7235=CARTESIAN_POINT ( 'NONE',  ( 1.687505431895960050E-16, 0.07874015748031508444, 1.377952755905512472 ) ) ;
#7258=CYLINDRICAL_SURFACE ( 'NONE', #20200, 0.2952755905511805778 ) ;
#7266=VECTOR ( 'NONE', #3866, 39.37007874015748143 ) ;
#7308=DIRECTION ( 'NONE',  ( 0.000000000000000000, 0.000000000000000000, -1.000000000000000000 ) ) ;
#7316=AXIS2_PLACEMENT_3D ( 'NONE', #16348, #706, #20055 ) ;
#7324=CARTESIAN_POINT ( 'NONE',  ( -2.073220866141732523E-16, 0.07874015748031495954, 1.692913385826771533 ) ) ;
#7349=DIRECTION ( 'NONE',  ( 0.000000000000000000, 0.000000000000000000, -1.000000000000000000 ) ) ;
#7367=AXIS2_PLACEMENT_3D ( 'NONE', #6849, #15477, #4714 ) ;
#7382=EDGE_CURVE ( 'NONE', #247, #1086, #6803, .T. ) ;
#7403=CARTESIAN_POINT ( 'NONE',  ( -1.197070535079588716, 0.4724409448818898127, -1.197070535079588716 ) ) ;
#7432=CARTESIAN_POINT ( 'NONE',  ( 2.531258147843938596E-16, 0.3937007873309092409, 2.066929133858267598 ) ) ;
#7459=VERTEX_POINT ( 'NONE', #7432 ) ;
#7465=ORIENTED_EDGE ( 'NONE', *, *, #15595, .F. ) ;
#7475=CARTESIAN_POINT ( 'NONE',  ( -2.073220866141732523E-16, 0.07874015748031491790, 1.692913385826771533 ) ) ;
#7487=DIRECTION ( 'NONE',  ( -0.000000000000000000, -1.000000000000000000, -0.000000000000000000 ) ) ;
#7495=ORIENTED_EDGE ( 'NONE', *, *, #15197, .T. ) ;
#7501=DIRECTION ( 'NONE',  ( 0.000000000000000000, 0.7071067805519554161, 0.7071067818211396183 ) ) ;
#7544=DIRECTION ( 'NONE',  ( 0.000000000000000000, 0.000000000000000000, -1.000000000000000000 ) ) ;
#7550=ORIENTED_EDGE ( 'NONE', *, *, #7382, .T. ) ;
#7555=ORIENTED_EDGE ( 'NONE', *, *, #15537, .F. ) ;
#7578=VECTOR ( 'NONE', #3479, 39.37007874015748143 ) ;
#7586=EDGE_CURVE ( 'NONE', #26351, #1498, #17633, .T. ) ;
#7590=VECTOR ( 'NONE', #24721, 39.37007874015748143 ) ;
#7608=ORIENTED_EDGE ( 'NONE', *, *, #17689, .T. ) ;
#7615=VERTEX_POINT ( 'NONE', #27080 ) ;
#7629=AXIS2_PLACEMENT_3D ( 'NONE', #22568, #14093, #7308 ) ;
#7643=VECTOR ( 'NONE', #14343, 39.37007874015748143 ) ;
#7669=ADVANCED_FACE ( 'NONE', ( #17313, #23686 ), #12924, .F. ) ;
#7677=CARTESIAN_POINT ( 'NONE',  ( -1.197070535079588716, 0.07874015748031491790, -1.197070535079588716 ) ) ;
#7681=CARTESIAN_POINT ( 'NONE',  ( 0.3937007874015748254, 0.9055118110236221041, 0.000000000000000000 ) ) ;
#7699=CARTESIAN_POINT ( 'NONE',  ( 1.687505431895960050E-16, 0.3543307086614172485, -1.377952755905512472 ) ) ;
#7703=VERTEX_POINT ( 'NONE', #21696 ) ;
#7711=CARTESIAN_POINT ( 'NONE',  ( 0.000000000000000000, 0.5905511811023621549, -0.3937007874015748254 ) ) ;
#7721=DIRECTION ( 'NONE',  ( 0.000000000000000000, 0.000000000000000000, 1.000000000000000000 ) ) ;
#7725=ORIENTED_EDGE ( 'NONE', *, *, #27857, .F. ) ;
#7750=ORIENTED_EDGE ( 'NONE', *, *, #12547, .F. ) ;
#7766=EDGE_CURVE ( 'NONE', #21688, #152, #2194, .T. ) ;
#7796=ORIENTED_EDGE ( 'NONE', *, *, #12460, .T. ) ;
#7802=CIRCLE ( 'NONE', #10944, 0.1181102362204720091 ) ;
#7817=CARTESIAN_POINT ( 'NONE',  ( 0.000000000000000000, 0.1968503937007875237, 0.000000000000000000 ) ) ;
#7821=EDGE_LOOP ( 'NONE', ( #5092, #5307 ) ) ;
#7827=LINE ( 'NONE', #22233, #27825 ) ;
#7832=ORIENTED_EDGE ( 'NONE', *, *, #709, .T. ) ;
#7859=ADVANCED_FACE ( 'NONE', ( #4718 ), #4994, .F. ) ;
#7874=DIRECTION ( 'NONE',  ( -0.000000000000000000, -1.000000000000000000, -0.000000000000000000 ) ) ;
#7893=ADVANCED_FACE ( 'NONE', ( #26334 ), #6995, .F. ) ;
#7901=CYLINDRICAL_SURFACE ( 'NONE', #6839, 0.1181102362204718703 ) ;
#7914=CARTESIAN_POINT ( 'NONE',  ( 0.000000000000000000, 0.3937007873309092409, -2.066929133858267598 ) ) ;
#7922=ORIENTED_EDGE ( 'NONE', *, *, #20571, .F. ) ;
#7923=DIRECTION ( 'NONE',  ( 1.000000000000000000, 0.000000000000000000, 0.000000000000000000 ) ) ;
#7926=ORIENTED_EDGE ( 'NONE', *, *, #15699, .T. ) ;
#7932=VERTEX_POINT ( 'NONE', #11091 ) ;
#7948=CYLINDRICAL_SURFACE ( 'NONE', #3055, 0.4921259842519685179 ) ;
#7950=DIRECTION ( 'NONE',  ( -0.000000000000000000, -1.000000000000000000, -0.000000000000000000 ) ) ;
#7951=EDGE_LOOP ( 'NONE', ( #1824, #14345 ) ) ;
#7990=PRODUCT_CONTEXT ( 'NONE', #2576, 'mechanical' ) ;
#8009=CARTESIAN_POINT ( 'NONE',  ( -1.197070535079588716, 0.4724409448818898127, -1.197070535079588716 ) ) ;
#8028=AXIS2_PLACEMENT_3D ( 'NONE', #13458, #5116, #9209 ) ;
#8066=DIRECTION ( 'NONE',  ( 0.000000000000000000, 0.000000000000000000, -1.000000000000000000 ) ) ;
#8077=CARTESIAN_POINT ( 'NONE',  ( 0.000000000000000000, 0.03937007874015751446, 0.000000000000000000 ) ) ;
#8118=VECTOR ( 'NONE', #7048, 39.37007874015748854 ) ;
#8160=EDGE_CURVE ( 'NONE', #3201, #12475, #23519, .T. ) ;
#8178=CARTESIAN_POINT ( 'NONE',  ( 4.821444091131312140E-17, 0.8661417322803149910, 0.3937007874015748254 ) ) ;
#8180=ORIENTED_EDGE ( 'NONE', *, *, #8214, .F. ) ;
#8192=CARTESIAN_POINT ( 'NONE',  ( 4.821444091131312140E-17, 0.5905511811023621549, 0.3937007874015748254 ) ) ;
#8214=EDGE_CURVE ( 'NONE', #21688, #16430, #5025, .T. ) ;
#8229=ORIENTED_EDGE ( 'NONE', *, *, #12797, .F. ) ;
#8244=CARTESIAN_POINT ( 'NONE',  ( 0.000000000000000000, 0.07874015748662489822, -0.2952755905511805778 ) ) ;
#8250=AXIS2_PLACEMENT_3D ( 'NONE', #19701, #24340, #2851 ) ;
#8259=ADVANCED_FACE ( 'NONE', ( #27115 ), #7901, .F. ) ;
#8276=CARTESIAN_POINT ( 'NONE',  ( 0.000000000000000000, 0.4724409448818898127, 0.000000000000000000 ) ) ;
#8294=AXIS2_PLACEMENT_3D ( 'NONE', #5257, #16145, #9626 ) ;
#8335=AXIS2_PLACEMENT_3D ( 'NONE', #16519, #3513, #1405 ) ;
#8345=CARTESIAN_POINT ( 'NONE',  ( 4.821444091131312140E-17, 0.8661417322803149910, 0.3937007874015748254 ) ) ;
#8362=CIRCLE ( 'NONE', #25940, 0.4921259842519685179 ) ;
#8372=EDGE_CURVE ( 'NONE', #19458, #23913, #12253, .T. ) ;
#8396=PLANE ( 'NONE',  #5082 ) ;
#8406=DIRECTION ( 'NONE',  ( 3.169619147893091460E-17, -0.9659258263664933786, 0.2588190448135661570 ) ) ;
#8426=CARTESIAN_POINT ( 'NONE',  ( 2.483043706975895149E-16, 0.4724409448818898127, 1.988188976448617584 ) ) ;
#8431=FACE_OUTER_BOUND ( 'NONE', #11310, .T. ) ;
#8446=ORIENTED_EDGE ( 'NONE', *, *, #22416, .T. ) ;
#8449=ORIENTED_EDGE ( 'NONE', *, *, #2784, .F. ) ;
#8450=DIRECTION ( 'NONE',  ( -0.000000000000000000, 1.000000000000000000, 0.000000000000000000 ) ) ;
#8455=( GEOMETRIC_REPRESENTATION_CONTEXT ( 3 ) GLOBAL_UNCERTAINTY_ASSIGNED_CONTEXT ( ( #857 ) ) GLOBAL_UNIT_ASSIGNED_CONTEXT ( ( #18780, #18205, #15975 ) ) REPRESENTATION_CONTEXT ( 'NONE', 'WORKASPACE' ) ) ;
#8461=ADVANCED_FACE ( 'NONE', ( #24908 ), #16873, .T. ) ;
#8477=ADVANCED_FACE ( 'NONE', ( #3716 ), #2772, .T. ) ;
#8498=CARTESIAN_POINT ( 'NONE',  ( 0.000000000000000000, 0.4724409448818898127, 0.000000000000000000 ) ) ;
#8507=EDGE_LOOP ( 'NONE', ( #20510, #14361, #9125, #2718 ) ) ;
#8513=FACE_BOUND ( 'NONE', #2970, .T. ) ;
#8529=EDGE_CURVE ( 'NONE', #13707, #12080, #15855, .T. ) ;
#8552=EDGE_CURVE ( 'NONE', #14474, #14467, #17557, .T. ) ;
#8590=FACE_OUTER_BOUND ( 'NONE', #13893, .T. ) ;
#8591=VERTEX_POINT ( 'NONE', #25620 ) ;
#8594=DIRECTION ( 'NONE',  ( 0.000000000000000000, 1.000000000000000000, 0.000000000000000000 ) ) ;
#8606=DIRECTION ( 'NONE',  ( 0.000000000000000000, 0.000000000000000000, -1.000000000000000000 ) ) ;
#8621=ORIENTED_EDGE ( 'NONE', *, *, #22494, .F. ) ;
#8659=CYLINDRICAL_SURFACE ( 'NONE', #22247, 1.377952755905512472 ) ;
#8703=CARTESIAN_POINT ( 'NONE',  ( 1.692913385826771533, 0.07874015748031495954, 3.109831496062992451E-16 ) ) ;
#8713=VERTEX_POINT ( 'NONE', #12591 ) ;
#8729=VERTEX_POINT ( 'NONE', #27008 ) ;
#8786=ORIENTED_EDGE ( 'NONE', *, *, #11893, .F. ) ;
#8822=ORIENTED_EDGE ( 'NONE', *, *, #23952, .T. ) ;
#8827=CARTESIAN_POINT ( 'NONE',  ( 1.687505431895960050E-16, 0.07874015748031495954, 1.377952755905512472 ) ) ;
#8883=DIRECTION ( 'NONE',  ( -0.000000000000000000, 1.000000000000000000, -0.000000000000000000 ) ) ;
#8960=CARTESIAN_POINT ( 'NONE',  ( 1.197070535079588716, 0.07874015748031495954, 1.197070535079588716 ) ) ;
#8968=ORIENTED_EDGE ( 'NONE', *, *, #10873, .F. ) ;
#9000=DIRECTION ( 'NONE',  ( -0.000000000000000000, 1.000000000000000000, 0.000000000000000000 ) ) ;
#9022=CARTESIAN_POINT ( 'NONE',  ( -1.692913385826771533, 0.07874015748031491790, -1.036610629921259805E-16 ) ) ;
#9034=LINE ( 'NONE', #11710, #25362 ) ;
#9051=EDGE_CURVE ( 'NONE', #25393, #11604, #15026, .T. ) ;
#9064=DIRECTION ( 'NONE',  ( -0.000000000000000000, 1.000000000000000000, -0.000000000000000000 ) ) ;
#9093=VECTOR ( 'NONE', #15177, 39.37007874015748143 ) ;
#9097=CARTESIAN_POINT ( 'NONE',  ( -2.073220866141732523E-16, 0.07874015748031491790, 1.574803149606299524 ) ) ;
#9101=EDGE_CURVE ( 'NONE', #7057, #1086, #9034, .T. ) ;
#9125=ORIENTED_EDGE ( 'NONE', *, *, #4983, .T. ) ;
#9148=AXIS2_PLACEMENT_3D ( 'NONE', #12266, #8450, #5926 ) ;
#9154=CIRCLE ( 'NONE', #24494, 0.1181102362204720091 ) ;
#9171=EDGE_CURVE ( 'NONE', #25145, #6614, #164, .T. ) ;
#9173=CARTESIAN_POINT ( 'NONE',  ( 0.000000000000000000, 0.8661417322803149910, 0.000000000000000000 ) ) ;
#9184=EDGE_LOOP ( 'NONE', ( #8786, #18721 ) ) ;
#9196=CIRCLE ( 'NONE', #4269, 0.2952755905511805778 ) ;
#9197=ORIENTED_EDGE ( 'NONE', *, *, #16116, .F. ) ;
#9209=DIRECTION ( 'NONE',  ( 0.000000000000000000, 0.000000000000000000, 1.000000000000000000 ) ) ;
#9214=FACE_OUTER_BOUND ( 'NONE', #21386, .T. ) ;
#9257=EDGE_CURVE ( 'NONE', #27168, #14000, #27400, .T. ) ;
#9269=AXIS2_PLACEMENT_3D ( 'NONE', #7324, #694, #2527 ) ;
#9272=CARTESIAN_POINT ( 'NONE',  ( -1.197070535079588716, 0.07874015748031491790, 1.078960298859116707 ) ) ;
#9296=DIRECTION ( 'NONE',  ( 0.000000000000000000, 0.000000000000000000, -1.000000000000000000 ) ) ;
#9302=DIRECTION ( 'NONE',  ( 0.000000000000000000, -1.000000000000000000, 0.000000000000000000 ) ) ;
#9310=DIRECTION ( 'NONE',  ( 0.000000000000000000, 0.000000000000000000, -1.000000000000000000 ) ) ;
#9341=DIRECTION ( 'NONE',  ( 0.000000000000000000, 0.000000000000000000, -1.000000000000000000 ) ) ;
#9373=CIRCLE ( 'NONE', #25175, 0.1181102362204718703 ) ;
#9388=ORIENTED_EDGE ( 'NONE', *, *, #13013, .F. ) ;
#9389=ORIENTED_EDGE ( 'NONE', *, *, #16116, .T. ) ;
#9427=DIRECTION ( 'NONE',  ( -0.000000000000000000, -1.000000000000000000, -0.000000000000000000 ) ) ;
#9428=VERTEX_POINT ( 'NONE', #7699 ) ;
#9441=CARTESIAN_POINT ( 'NONE',  ( 0.000000000000000000, -1.533249767903113305E-16, 0.000000000000000000 ) ) ;
#9449=DIRECTION ( 'NONE',  ( 0.000000000000000000, -0.000000000000000000, -1.000000000000000000 ) ) ;
#9455=CARTESIAN_POINT ( 'NONE',  ( 0.000000000000000000, 0.03937007874015751446, 0.000000000000000000 ) ) ;
#9482=EDGE_CURVE ( 'NONE', #13627, #3934, #27049, .T. ) ;
#9490=ORIENTED_EDGE ( 'NONE', *, *, #14990, .F. ) ;
#9513=ADVANCED_FACE ( 'NONE', ( #25487, #27611 ), #8396, .T. ) ;
#9516=VECTOR ( 'NONE', #8406, 39.37007874015748854 ) ;
#9530=EDGE_LOOP ( 'NONE', ( #21260, #6337, #21119, #291 ) ) ;
#9592=DIRECTION ( 'NONE',  ( 0.000000000000000000, 0.000000000000000000, -1.000000000000000000 ) ) ;
#9596=AXIS2_PLACEMENT_3D ( 'NONE', #20645, #23354, #1298 ) ;
#9618=ORIENTED_EDGE ( 'NONE', *, *, #11461, .T. ) ;
#9626=DIRECTION ( 'NONE',  ( 0.000000000000000000, 0.000000000000000000, 1.000000000000000000 ) ) ;
#9638=CIRCLE ( 'NONE', #26851, 1.377952755905512472 ) ;
#9643=EDGE_LOOP ( 'NONE', ( #8449, #6690, #6206, #22522 ) ) ;
#9645=CIRCLE ( 'NONE', #17325, 0.1181102362204720091 ) ;
#9651=AXIS2_PLACEMENT_3D ( 'NONE', #2102, #12423, #10715 ) ;
#9668=AXIS2_PLACEMENT_3D ( 'NONE', #1003, #13849, #27133 ) ;
#9681=VECTOR ( 'NONE', #12940, 39.37007874015748143 ) ;
#9688=EDGE_LOOP ( 'NONE', ( #6476, #406, #24034, #9197 ) ) ;
#9689=EDGE_LOOP ( 'NONE', ( #16489, #870, #20492, #16523 ) ) ;
#9691=DIRECTION ( 'NONE',  ( 0.000000000000000000, 0.000000000000000000, -1.000000000000000000 ) ) ;
#9721=ORIENTED_EDGE ( 'NONE', *, *, #13412, .F. ) ;
#9727=ADVANCED_FACE ( 'NONE', ( #17145 ), #8659, .F. ) ;
#9790=CARTESIAN_POINT ( 'NONE',  ( 1.692913385826771533, 0.07874015748031491790, 3.109831496062992451E-16 ) ) ;
#9825=DIRECTION ( 'NONE',  ( -0.000000000000000000, 1.000000000000000000, -0.000000000000000000 ) ) ;
#9832=DIRECTION ( 'NONE',  ( -0.000000000000000000, -1.000000000000000000, -0.000000000000000000 ) ) ;
#9866=ORIENTED_EDGE ( 'NONE', *, *, #15668, .F. ) ;
#9880=VERTEX_POINT ( 'NONE', #26856 ) ;
#9888=CIRCLE ( 'NONE', #16389, 0.7874015748031496509 ) ;
#9899=CYLINDRICAL_SURFACE ( 'NONE', #13742, 0.3937007874015748254 ) ;
#9900=CARTESIAN_POINT ( 'NONE',  ( 0.000000000000000000, 0.1968503937007875237, -1.377952755905512472 ) ) ;
#9963=CARTESIAN_POINT ( 'NONE',  ( -1.197070535079588716, 0.07874015748031491790, 1.197070535079588716 ) ) ;
#9967=ORIENTED_EDGE ( 'NONE', *, *, #25976, .T. ) ;
#9999=ORIENTED_EDGE ( 'NONE', *, *, #24672, .T. ) ;
#10033=CARTESIAN_POINT ( 'NONE',  ( 0.000000000000000000, 0.3543307086614173040, 0.000000000000000000 ) ) ;
#10062=DIRECTION ( 'NONE',  ( 0.000000000000000000, 0.000000000000000000, -1.000000000000000000 ) ) ;
#10071=EDGE_CURVE ( 'NONE', #11604, #25393, #9154, .T. ) ;
#10104=CARTESIAN_POINT ( 'NONE',  ( -1.197070535079588716, 0.07874015748031495954, 1.078960298859116707 ) ) ;
#10110=DIRECTION ( 'NONE',  ( 0.000000000000000000, 0.000000000000000000, 1.000000000000000000 ) ) ;
#10156=CARTESIAN_POINT ( 'NONE',  ( 0.000000000000000000, 0.9055118110236221041, 0.000000000000000000 ) ) ;
#10160=ADVANCED_FACE ( 'NONE', ( #5824 ), #3680, .F. ) ;
#10167=ORIENTED_EDGE ( 'NONE', *, *, #14778, .F. ) ;
#10187=CARTESIAN_POINT ( 'NONE',  ( 1.692913385826771533, 0.4724409448818898127, -0.1181102362204716899 ) ) ;
#10195=DIRECTION ( 'NONE',  ( 0.000000000000000000, 0.000000000000000000, -1.000000000000000000 ) ) ;
#10207=EDGE_LOOP ( 'NONE', ( #12640, #5563, #7550, #10492 ) ) ;
#10246=DIRECTION ( 'NONE',  ( 0.000000000000000000, 0.000000000000000000, -1.000000000000000000 ) ) ;
#10264=EDGE_CURVE ( 'NONE', #3934, #24215, #2794, .T. ) ;
#10268=VERTEX_POINT ( 'NONE', #18639 ) ;
#10293=AXIS2_PLACEMENT_3D ( 'NONE', #19230, #27862, #25874 ) ;
#10310=DIRECTION ( 'NONE',  ( 0.000000000000000000, 0.000000000000000000, -1.000000000000000000 ) ) ;
#10326=AXIS2_PLACEMENT_3D ( 'NONE', #24650, #22832, #7721 ) ;
#10386=CARTESIAN_POINT ( 'NONE',  ( -1.692913385826771533, 0.07874015748031495954, 0.1181102362204718981 ) ) ;
#10389=CYLINDRICAL_SURFACE ( 'NONE', #6702, 0.7874015748208159637 ) ;
#10402=CYLINDRICAL_SURFACE ( 'NONE', #27867, 0.7874015748208159637 ) ;
#10407=LINE ( 'NONE', #17191, #9681 ) ;
#10430=CARTESIAN_POINT ( 'NONE',  ( -1.197070535079588716, 0.07874015748031495954, 1.197070535079588716 ) ) ;
#10449=EDGE_LOOP ( 'NONE', ( #21860, #13923, #1184, #3638 ) ) ;
#10465=DIRECTION ( 'NONE',  ( -0.000000000000000000, -1.000000000000000000, -0.000000000000000000 ) ) ;
#10492=ORIENTED_EDGE ( 'NONE', *, *, #4983, .F. ) ;
#10497=ORIENTED_EDGE ( 'NONE', *, *, #19993, .T. ) ;
#10531=DIRECTION ( 'NONE',  ( 0.000000000000000000, -0.000000000000000000, 1.000000000000000000 ) ) ;
#10536=DIRECTION ( 'NONE',  ( 0.000000000000000000, -0.000000000000000000, -1.000000000000000000 ) ) ;
#10560=DIRECTION ( 'NONE',  ( 0.000000000000000000, 0.000000000000000000, 1.000000000000000000 ) ) ;
#10580=AXIS2_PLACEMENT_3D ( 'NONE', #12013, #11585, #9592 ) ;
#10592=EDGE_CURVE ( 'NONE', #1086, #247, #10925, .T. ) ;
#10596=CARTESIAN_POINT ( 'NONE',  ( 0.000000000000000000, 0.4724409448818898127, 0.000000000000000000 ) ) ;
#10617=ORIENTED_EDGE ( 'NONE', *, *, #11897, .F. ) ;
#10623=FACE_BOUND ( 'NONE', #25852, .T. ) ;
#10642=EDGE_CURVE ( 'NONE', #24215, #3934, #3695, .T. ) ;
#10664=ORIENTED_EDGE ( 'NONE', *, *, #5649, .F. ) ;
#10688=DIRECTION ( 'NONE',  ( 0.000000000000000000, 0.000000000000000000, -1.000000000000000000 ) ) ;
#10715=DIRECTION ( 'NONE',  ( 0.000000000000000000, 0.000000000000000000, -1.000000000000000000 ) ) ;
#10731=CARTESIAN_POINT ( 'NONE',  ( 0.000000000000000000, 0.8661417322803149910, 0.000000000000000000 ) ) ;
#10745=DIRECTION ( 'NONE',  ( 0.000000000000000000, 0.000000000000000000, 1.000000000000000000 ) ) ;
#10784=DIRECTION ( 'NONE',  ( 0.000000000000000000, 0.000000000000000000, -1.000000000000000000 ) ) ;
#10810=CYLINDRICAL_SURFACE ( 'NONE', #18894, 1.377952755905512472 ) ;
#10819=( NAMED_UNIT ( * ) SI_UNIT ( $, .STERADIAN. ) SOLID_ANGLE_UNIT ( ) ) ;
#10822=EDGE_CURVE ( 'NONE', #13016, #2225, #5594, .T. ) ;
#10840=ORIENTED_EDGE ( 'NONE', *, *, #8552, .T. ) ;
#10848=VERTEX_POINT ( 'NONE', #23541 ) ;
#10873=EDGE_CURVE ( 'NONE', #25509, #16023, #12291, .T. ) ;
#10925=CIRCLE ( 'NONE', #14630, 2.066929133858267598 ) ;
#10937=ADVANCED_FACE ( 'NONE', ( #2314 ), #11354, .F. ) ;
#10944=AXIS2_PLACEMENT_3D ( 'NONE', #9790, #14038, #10062 ) ;
#10965=ORIENTED_EDGE ( 'NONE', *, *, #10071, .T. ) ;
#10972=ORIENTED_EDGE ( 'NONE', *, *, #6835, .T. ) ;
#10978=CARTESIAN_POINT ( 'NONE',  ( -1.197070535079588716, 0.4724409448818898127, 1.078960298859116707 ) ) ;
#10998=FACE_BOUND ( 'NONE', #7821, .T. ) ;
#11011=CARTESIAN_POINT ( 'NONE',  ( 0.000000000000000000, 0.03937007874015751446, 0.5511811023975373702 ) ) ;
#11019=AXIS2_PLACEMENT_3D ( 'NONE', #18733, #7874, #5762 ) ;
#11034=EDGE_CURVE ( 'NONE', #12707, #10268, #7802, .T. ) ;
#11063=DIRECTION ( 'NONE',  ( -0.000000000000000000, 1.000000000000000000, -0.000000000000000000 ) ) ;
#11084=ORIENTED_EDGE ( 'NONE', *, *, #4876, .F. ) ;
#11091=CARTESIAN_POINT ( 'NONE',  ( 0.000000000000000000, 0.07874015748662489822, -0.2952755905511805778 ) ) ;
#11106=DIRECTION ( 'NONE',  ( 0.000000000000000000, 0.000000000000000000, -1.000000000000000000 ) ) ;
#11109=ORIENTED_EDGE ( 'NONE', *, *, #114, .F. ) ;
#11133=AXIS2_PLACEMENT_3D ( 'NONE', #27672, #14703, #25827 ) ;
#11136=EDGE_CURVE ( 'NONE', #7703, #2225, #17266, .T. ) ;
#11190=CARTESIAN_POINT ( 'NONE',  ( -2.073220866141732523E-16, 0.4724409448818898127, 1.692913385826771533 ) ) ;
#11226=DIRECTION ( 'NONE',  ( -0.000000000000000000, -1.000000000000000000, -0.000000000000000000 ) ) ;
#11260=EDGE_LOOP ( 'NONE', ( #25316, #20948 ) ) ;
#11270=VECTOR ( 'NONE', #3000, 39.37007874015748143 ) ;
#11305=CARTESIAN_POINT ( 'NONE',  ( 0.000000000000000000, 0.9055118110236221041, 0.000000000000000000 ) ) ;
#11310=EDGE_LOOP ( 'NONE', ( #26782, #13570, #21617, #25623 ) ) ;
#11313=ORIENTED_EDGE ( 'NONE', *, *, #27668, .T. ) ;
#11344=ORIENTED_EDGE ( 'NONE', *, *, #2784, .T. ) ;
#11354=CYLINDRICAL_SURFACE ( 'NONE', #8250, 0.1181102362204720091 ) ;
#11385=CARTESIAN_POINT ( 'NONE',  ( 0.000000000000000000, 0.1574803148899641958, 0.000000000000000000 ) ) ;
#11416=CIRCLE ( 'NONE', #27675, 1.377952755905512472 ) ;
#11427=ADVANCED_FACE ( 'NONE', ( #8590, #25121, #12554, #6342, #16653, #1672, #1813, #25263, #14971, #23018 ), #14704, .T. ) ;
#11447=FACE_OUTER_BOUND ( 'NONE', #27179, .T. ) ;
#11461=EDGE_CURVE ( 'NONE', #9428, #13016, #11416, .T. ) ;
#11465=AXIS2_PLACEMENT_3D ( 'NONE', #10731, #44, #8606 ) ;
#11469=ORIENTED_EDGE ( 'NONE', *, *, #22166, .F. ) ;
#11476=DIRECTION ( 'NONE',  ( 0.000000000000000000, 0.000000000000000000, -1.000000000000000000 ) ) ;
#11483=CARTESIAN_POINT ( 'NONE',  ( 0.000000000000000000, 0.000000000000000000, -0.2952755905511805778 ) ) ;
#11486=AXIS2_PLACEMENT_3D ( 'NONE', #14284, #22895, #12143 ) ;
#11507=FACE_OUTER_BOUND ( 'NONE', #3068, .T. ) ;
#11515=DIRECTION ( 'NONE',  ( 0.000000000000000000, 0.000000000000000000, 1.000000000000000000 ) ) ;
#11526=DIRECTION ( 'NONE',  ( -0.000000000000000000, -1.000000000000000000, -0.000000000000000000 ) ) ;
#11536=CARTESIAN_POINT ( 'NONE',  ( 0.000000000000000000, 0.4724409448818898127, 0.000000000000000000 ) ) ;
#11583=CARTESIAN_POINT ( 'NONE',  ( -1.197070535079588716, 0.07874015748031491790, 1.197070535079588716 ) ) ;
#11585=DIRECTION ( 'NONE',  ( 0.000000000000000000, -1.000000000000000000, 0.000000000000000000 ) ) ;
#11588=AXIS2_PLACEMENT_3D ( 'NONE', #5229, #3665, #7923 ) ;
#11595=EDGE_LOOP ( 'NONE', ( #17928, #17734 ) ) ;
#11601=DIRECTION ( 'NONE',  ( -0.000000000000000000, -1.000000000000000000, -0.000000000000000000 ) ) ;
#11604=VERTEX_POINT ( 'NONE', #21588 ) ;
#11605=AXIS2_PLACEMENT_3D ( 'NONE', #23955, #4588, #26755 ) ;
#11615=LINE ( 'NONE', #22777, #3846 ) ;
#11620=CARTESIAN_POINT ( 'NONE',  ( -1.692913385826771533, 0.07874015748031491790, -0.1181102362204721062 ) ) ;
#11637=CARTESIAN_POINT ( 'NONE',  ( 0.000000000000000000, 0.000000000000000000, 0.000000000000000000 ) ) ;
#11679=FACE_OUTER_BOUND ( 'NONE', #18129, .T. ) ;
#11710=CARTESIAN_POINT ( 'NONE',  ( 2.434829265934773153E-16, 0.07874015748031495954, -1.988188976307287970 ) ) ;
#11713=CIRCLE ( 'NONE', #22544, 0.1181102362204720091 ) ;
#11745=ORIENTED_EDGE ( 'NONE', *, *, #14857, .F. ) ;
#11751=LINE ( 'NONE', #22633, #12095 ) ;
#11774=LINE ( 'NONE', #20392, #3551 ) ;
#11782=ORIENTED_EDGE ( 'NONE', *, *, #9257, .F. ) ;
#11785=EDGE_LOOP ( 'NONE', ( #11109, #19027 ) ) ;
#11805=AXIS2_PLACEMENT_3D ( 'NONE', #25052, #6145, #14332 ) ;
#11806=EDGE_LOOP ( 'NONE', ( #3946, #18936, #2135, #18787 ) ) ;
#11837=ORIENTED_EDGE ( 'NONE', *, *, #25230, .F. ) ;
#11851=CARTESIAN_POINT ( 'NONE',  ( 4.821444091131312140E-17, 0.9055118110236221041, 0.3937007874015748254 ) ) ;
#11871=SHAPE_REPRESENTATION_RELATIONSHIP ( 'NONE' , 'NONE' ,  #4612, #3606 ) ;
#11893=EDGE_CURVE ( 'NONE', #15321, #8729, #13544, .T. ) ;
#11897=EDGE_CURVE ( 'NONE', #14000, #12475, #3618, .T. ) ;
#11898=AXIS2_PLACEMENT_3D ( 'NONE', #26686, #20625, #15967 ) ;
#11945=ADVANCED_FACE ( 'NONE', ( #12514 ), #21130, .F. ) ;
#11979=EDGE_CURVE ( 'NONE', #25145, #7459, #3544, .T. ) ;
#11993=VERTEX_POINT ( 'NONE', #1178 ) ;
#12003=AXIS2_PLACEMENT_3D ( 'NONE', #20042, #9427, #26392 ) ;
#12013=CARTESIAN_POINT ( 'NONE',  ( 0.000000000000000000, 0.9055118110236221041, 0.000000000000000000 ) ) ;
#12054=ORIENTED_EDGE ( 'NONE', *, *, #27465, .F. ) ;
#12080=VERTEX_POINT ( 'NONE', #10187 ) ;
#12094=CIRCLE ( 'NONE', #13002, 0.1181102362204720091 ) ;
#12095=VECTOR ( 'NONE', #892, 39.37007874015748143 ) ;
#12116=AXIS2_PLACEMENT_3D ( 'NONE', #17290, #19823, #26316 ) ;
#12143=DIRECTION ( 'NONE',  ( 0.000000000000000000, 0.000000000000000000, -1.000000000000000000 ) ) ;
#12152=DIRECTION ( 'NONE',  ( 0.000000000000000000, 0.000000000000000000, -1.000000000000000000 ) ) ;
#12187=CARTESIAN_POINT ( 'NONE',  ( 6.026805113914139867E-17, 0.4724409448818898127, 0.4921259842519685179 ) ) ;
#12193=DIRECTION ( 'NONE',  ( 0.000000000000000000, -1.000000000000000000, 0.000000000000000000 ) ) ;
#12216=LINE ( 'NONE', #16735, #9516 ) ;
#12247=LINE ( 'NONE', #16356, #7578 ) ;
#12253=CIRCLE ( 'NONE', #529, 0.1181102362204718703 ) ;
#12263=ORIENTED_EDGE ( 'NONE', *, *, #14355, .F. ) ;
#12266=CARTESIAN_POINT ( 'NONE',  ( 2.066929133858267598, 0.4724409448818898127, 0.000000000000000000 ) ) ;
#12291=CIRCLE ( 'NONE', #1930, 0.4921259842519685179 ) ;
#12311=DIRECTION ( 'NONE',  ( 0.000000000000000000, 0.000000000000000000, -1.000000000000000000 ) ) ;
#12316=DIRECTION ( 'NONE',  ( 0.000000000000000000, 0.000000000000000000, -1.000000000000000000 ) ) ;
#12353=CARTESIAN_POINT ( 'NONE',  ( 0.000000000000000000, 0.07874015748031495954, -1.377952755905512472 ) ) ;
#12360=AXIS2_PLACEMENT_3D ( 'NONE', #27589, #6531, #15161 ) ;
#12391=DIRECTION ( 'NONE',  ( 0.000000000000000000, 0.000000000000000000, -1.000000000000000000 ) ) ;
#12423=DIRECTION ( 'NONE',  ( 0.000000000000000000, -1.000000000000000000, 0.000000000000000000 ) ) ;
#12449=DIRECTION ( 'NONE',  ( 0.000000000000000000, 0.000000000000000000, -1.000000000000000000 ) ) ;
#12460=EDGE_CURVE ( 'NONE', #12934, #12849, #2741, .T. ) ;
#12475=VERTEX_POINT ( 'NONE', #7711 ) ;
#12497=VERTEX_POINT ( 'NONE', #21262 ) ;
#12501=CARTESIAN_POINT ( 'NONE',  ( 1.197070535079588716, 0.4724409448818898127, 1.078960298859116707 ) ) ;
#12514=FACE_OUTER_BOUND ( 'NONE', #24150, .T. ) ;
#12519=EDGE_CURVE ( 'NONE', #8591, #16564, #12216, .T. ) ;
#12537=DIRECTION ( 'NONE',  ( 0.000000000000000000, -1.000000000000000000, 0.000000000000000000 ) ) ;
#12547=EDGE_CURVE ( 'NONE', #1638, #17537, #1864, .T. ) ;
#12554=FACE_BOUND ( 'NONE', #7951, .T. ) ;
#12562=CYLINDRICAL_SURFACE ( 'NONE', #9651, 0.3937007874015748254 ) ;
#12564=VERTEX_POINT ( 'NONE', #12501 ) ;
#12591=CARTESIAN_POINT ( 'NONE',  ( 0.000000000000000000, -1.533249767903113305E-16, -0.3163739521363750362 ) ) ;
#12604=CARTESIAN_POINT ( 'NONE',  ( -1.197070535079588716, 0.4724409448818898127, -1.315180771300060503 ) ) ;
#12616=CARTESIAN_POINT ( 'NONE',  ( -2.073220866141732523E-16, 0.4724409448818898127, 1.574803149606299524 ) ) ;
#12628=CIRCLE ( 'NONE', #3122, 0.3163739521363750362 ) ;
#12630=ORIENTED_EDGE ( 'NONE', *, *, #10822, .T. ) ;
#12640=ORIENTED_EDGE ( 'NONE', *, *, #18523, .T. ) ;
#12652=EDGE_LOOP ( 'NONE', ( #8229, #2480, #27410, #14347 ) ) ;
#12672=DIRECTION ( 'NONE',  ( 0.000000000000000000, -1.000000000000000000, 0.000000000000000000 ) ) ;
#12674=ORIENTED_EDGE ( 'NONE', *, *, #21441, .F. ) ;
#12683=AXIS2_PLACEMENT_3D ( 'NONE', #8960, #15877, #17709 ) ;
#12707=VERTEX_POINT ( 'NONE', #22641 ) ;
#12708=DIRECTION ( 'NONE',  ( 0.000000000000000000, 0.000000000000000000, -1.000000000000000000 ) ) ;
#12736=EDGE_LOOP ( 'NONE', ( #320, #789 ) ) ;
#12751=DIRECTION ( 'NONE',  ( -0.000000000000000000, 1.000000000000000000, -0.000000000000000000 ) ) ;
#12767=ORIENTED_EDGE ( 'NONE', *, *, #14872, .F. ) ;
#12788=LINE ( 'NONE', #10104, #7165 ) ;
#12797=EDGE_CURVE ( 'NONE', #12849, #27168, #23184, .T. ) ;
#12818=AXIS2_PLACEMENT_3D ( 'NONE', #12875, #6806, #23908 ) ;
#12849=VERTEX_POINT ( 'NONE', #3815 ) ;
#12875=CARTESIAN_POINT ( 'NONE',  ( 0.000000000000000000, 0.8661417322803149910, 0.000000000000000000 ) ) ;
#12885=CARTESIAN_POINT ( 'NONE',  ( 0.000000000000000000, 0.07874015748031495954, 0.000000000000000000 ) ) ;
#12901=CARTESIAN_POINT ( 'NONE',  ( 0.000000000000000000, -1.533249767903113305E-16, 0.000000000000000000 ) ) ;
#12923=AXIS2_PLACEMENT_3D ( 'NONE', #19843, #17708, #26062 ) ;
#12924=PLANE ( 'NONE',  #4556 ) ;
#12925=CIRCLE ( 'NONE', #5729, 0.1181102362204720091 ) ;
#12934=VERTEX_POINT ( 'NONE', #14240 ) ;
#12940=DIRECTION ( 'NONE',  ( -0.000000000000000000, -1.000000000000000000, -0.000000000000000000 ) ) ;
#13002=AXIS2_PLACEMENT_3D ( 'NONE', #847, #24694, #20050 ) ;
#13006=LINE ( 'NONE', #19370, #17391 ) ;
#13008=CYLINDRICAL_SURFACE ( 'NONE', #19783, 0.1181102362204720091 ) ;
#13013=EDGE_CURVE ( 'NONE', #3201, #27168, #4161, .T. ) ;
#13016=VERTEX_POINT ( 'NONE', #3762 ) ;
#13034=AXIS2_PLACEMENT_3D ( 'NONE', #17239, #23748, #27210 ) ;
#13040=LINE ( 'NONE', #19811, #17571 ) ;
#13102=ORIENTED_EDGE ( 'NONE', *, *, #14275, .T. ) ;
#13116=ORIENTED_EDGE ( 'NONE', *, *, #15401, .T. ) ;
#13128=FACE_OUTER_BOUND ( 'NONE', #938, .T. ) ;
#13143=ADVANCED_FACE ( 'NONE', ( #4055 ), #2332, .F. ) ;
#13149=DIRECTION ( 'NONE',  ( -0.000000000000000000, -1.000000000000000000, -0.000000000000000000 ) ) ;
#13189=PRODUCT ( 'Index Plate', 'Index Plate', '', ( #7990 ) ) ;
#13209=EDGE_LOOP ( 'NONE', ( #5807, #10497, #16552, #17644 ) ) ;
#13217=CARTESIAN_POINT ( 'NONE',  ( 0.000000000000000000, -1.707404996040164512E-16, 0.000000000000000000 ) ) ;
#13220=DIRECTION ( 'NONE',  ( -0.000000000000000000, -1.000000000000000000, -0.000000000000000000 ) ) ;
#13231=DIRECTION ( 'NONE',  ( 0.000000000000000000, -1.000000000000000000, 0.000000000000000000 ) ) ;
#13234=ORIENTED_EDGE ( 'NONE', *, *, #19361, .T. ) ;
#13242=CIRCLE ( 'NONE', #7367, 0.5905511811200284678 ) ;
#13262=ORIENTED_EDGE ( 'NONE', *, *, #8372, .F. ) ;
#13264=CARTESIAN_POINT ( 'NONE',  ( -1.692913385826771533, 0.4724409448818898127, -1.036610629921259805E-16 ) ) ;
#13271=FACE_OUTER_BOUND ( 'NONE', #21293, .T. ) ;
#13291=DIRECTION ( 'NONE',  ( -0.000000000000000000, 1.000000000000000000, -0.000000000000000000 ) ) ;
#13313=DIRECTION ( 'NONE',  ( 0.000000000000000000, 0.000000000000000000, 1.000000000000000000 ) ) ;
#13349=DIRECTION ( 'NONE',  ( -0.000000000000000000, 1.000000000000000000, -0.000000000000000000 ) ) ;
#13366=DIRECTION ( 'NONE',  ( 0.000000000000000000, 1.000000000000000000, 0.000000000000000000 ) ) ;
#13373=CARTESIAN_POINT ( 'NONE',  ( -1.197070535079588716, 0.07874015748031495954, 1.197070535079588716 ) ) ;
#13408=DIRECTION ( 'NONE',  ( 0.000000000000000000, 0.000000000000000000, -1.000000000000000000 ) ) ;
#13412=EDGE_CURVE ( 'NONE', #17502, #22837, #21783, .T. ) ;
#13420=MECHANICAL_DESIGN_GEOMETRIC_PRESENTATION_REPRESENTATION('',(#3013),#2145);
#13423=CARTESIAN_POINT ( 'NONE',  ( 9.642888182478974314E-17, 0.1968503937007875237, 0.7874015748208159637 ) ) ;
#13434=VECTOR ( 'NONE', #5328, 39.37007874015748143 ) ;
#13443=AXIS2_PLACEMENT_3D ( 'NONE', #25005, #14737, #5669 ) ;
#13458=CARTESIAN_POINT ( 'NONE',  ( 1.692913385826771533, 0.4724409448818898127, 3.109831496062992451E-16 ) ) ;
#13470=CIRCLE ( 'NONE', #1310, 2.066929133858267598 ) ;
#13481=EDGE_LOOP ( 'NONE', ( #23542, #2898 ) ) ;
#13490=VERTEX_POINT ( 'NONE', #14457 ) ;
#13540=ORIENTED_EDGE ( 'NONE', *, *, #24173, .F. ) ;
#13544=CIRCLE ( 'NONE', #4974, 0.1181102362204720091 ) ;
#13546=LINE ( 'NONE', #2796, #21222 ) ;
#13556=PLANE ( 'NONE',  #20918 ) ;
#13570=ORIENTED_EDGE ( 'NONE', *, *, #26124, .T. ) ;
#13590=FACE_OUTER_BOUND ( 'NONE', #9643, .T. ) ;
#13600=EDGE_CURVE ( 'NONE', #12849, #12934, #22685, .T. ) ;
#13627=VERTEX_POINT ( 'NONE', #19662 ) ;
#13654=DIRECTION ( 'NONE',  ( 0.000000000000000000, 0.000000000000000000, 1.000000000000000000 ) ) ;
#13672=EDGE_CURVE ( 'NONE', #18301, #18986, #193, .T. ) ;
#13675=DIRECTION ( 'NONE',  ( 0.000000000000000000, 0.000000000000000000, 1.000000000000000000 ) ) ;
#13690=LINE ( 'NONE', #17905, #2060 ) ;
#13707=VERTEX_POINT ( 'NONE', #2543 ) ;
#13742=AXIS2_PLACEMENT_3D ( 'NONE', #23050, #6654, #26133 ) ;
#13747=DIRECTION ( 'NONE',  ( 0.000000000000000000, -1.000000000000000000, 0.000000000000000000 ) ) ;
#13768=VECTOR ( 'NONE', #23092, 39.37007874015748143 ) ;
#13829=ORIENTED_EDGE ( 'NONE', *, *, #27822, .F. ) ;
#13849=DIRECTION ( 'NONE',  ( -0.000000000000000000, 1.000000000000000000, -0.000000000000000000 ) ) ;
#13858=VERTEX_POINT ( 'NONE', #3223 ) ;
#13885=AXIS2_PLACEMENT_3D ( 'NONE', #3216, #4933, #7066 ) ;
#13893=EDGE_LOOP ( 'NONE', ( #11313, #17170 ) ) ;
#13923=ORIENTED_EDGE ( 'NONE', *, *, #1427, .T. ) ;
#13978=ORIENTED_EDGE ( 'NONE', *, *, #709, .F. ) ;
#13985=DIRECTION ( 'NONE',  ( 0.000000000000000000, 0.000000000000000000, -1.000000000000000000 ) ) ;
#14000=VERTEX_POINT ( 'NONE', #8192 ) ;
#14020=DIRECTION ( 'NONE',  ( 0.000000000000000000, 0.000000000000000000, 1.000000000000000000 ) ) ;
#14038=DIRECTION ( 'NONE',  ( -0.000000000000000000, -1.000000000000000000, -0.000000000000000000 ) ) ;
#14061=CARTESIAN_POINT ( 'NONE',  ( -1.197070535079588716, 0.07874015748031491790, -1.078960298859116707 ) ) ;
#14093=DIRECTION ( 'NONE',  ( -0.000000000000000000, -1.000000000000000000, -0.000000000000000000 ) ) ;
#14096=CARTESIAN_POINT ( 'NONE',  ( 0.000000000000000000, 0.07874015748031495954, 0.000000000000000000 ) ) ;
#14109=ORIENTED_EDGE ( 'NONE', *, *, #25627, .F. ) ;
#14123=DIRECTION ( 'NONE',  ( 0.000000000000000000, 0.000000000000000000, -1.000000000000000000 ) ) ;
#14146=AXIS2_PLACEMENT_3D ( 'NONE', #4405, #19513, #202 ) ;
#14180=DIRECTION ( 'NONE',  ( -0.000000000000000000, -1.000000000000000000, -0.000000000000000000 ) ) ;
#14195=CARTESIAN_POINT ( 'NONE',  ( 1.197070535079588716, 0.07874015748031495954, 1.078960298859116707 ) ) ;
#14200=DIRECTION ( 'NONE',  ( 0.000000000000000000, 0.000000000000000000, -1.000000000000000000 ) ) ;
#14231=ORIENTED_EDGE ( 'NONE', *, *, #14355, .T. ) ;
#14240=CARTESIAN_POINT ( 'NONE',  ( 0.000000000000000000, 0.9055118110236221041, -0.3831516066089791228 ) ) ;
#14248=CARTESIAN_POINT ( 'NONE',  ( 0.000000000000000000, 0.03937007874015747977, 0.000000000000000000 ) ) ;
#14272=DIRECTION ( 'NONE',  ( 0.000000000000000000, 0.000000000000000000, 1.000000000000000000 ) ) ;
#14275=EDGE_CURVE ( 'NONE', #24515, #25393, #26650, .T. ) ;
#14284=CARTESIAN_POINT ( 'NONE',  ( 0.000000000000000000, 0.000000000000000000, 0.000000000000000000 ) ) ;
#14290=AXIS2_PLACEMENT_3D ( 'NONE', #20393, #24763, #18251 ) ;
#14323=DIRECTION ( 'NONE',  ( 0.000000000000000000, 0.000000000000000000, 1.000000000000000000 ) ) ;
#14332=DIRECTION ( 'NONE',  ( 0.000000000000000000, 0.000000000000000000, 1.000000000000000000 ) ) ;
#14343=DIRECTION ( 'NONE',  ( -0.000000000000000000, -1.000000000000000000, -0.000000000000000000 ) ) ;
#14345=ORIENTED_EDGE ( 'NONE', *, *, #23172, .F. ) ;
#14346=ORIENTED_EDGE ( 'NONE', *, *, #20836, .T. ) ;
#14347=ORIENTED_EDGE ( 'NONE', *, *, #5192, .F. ) ;
#14348=PRODUCT_DEFINITION_FORMATION_WITH_SPECIFIED_SOURCE ( 'ANY', '', #13189, .NOT_KNOWN. ) ;
#14355=EDGE_CURVE ( 'NONE', #25308, #17724, #6049, .T. ) ;
#14361=ORIENTED_EDGE ( 'NONE', *, *, #298, .T. ) ;
#14365=DIRECTION ( 'NONE',  ( -0.000000000000000000, -1.000000000000000000, -0.000000000000000000 ) ) ;
#14388=CARTESIAN_POINT ( 'NONE',  ( 0.000000000000000000, 0.4724409448818898127, -1.988188976448617584 ) ) ;
#14394=CARTESIAN_POINT ( 'NONE',  ( 0.000000000000000000, 0.1968503937007875237, 0.000000000000000000 ) ) ;
#14400=CIRCLE ( 'NONE', #3530, 0.3937007874015748254 ) ;
#14431=EDGE_LOOP ( 'NONE', ( #23312, #15590, #17168, #9866 ) ) ;
#14442=FACE_OUTER_BOUND ( 'NONE', #27609, .T. ) ;
#14457=CARTESIAN_POINT ( 'NONE',  ( 0.000000000000000000, 0.5905511811023621549, -0.4921259842519685179 ) ) ;
#14460=CARTESIAN_POINT ( 'NONE',  ( 0.000000000000000000, 0.9055118110236221041, 0.000000000000000000 ) ) ;
#14467=VERTEX_POINT ( 'NONE', #4978 ) ;
#14474=VERTEX_POINT ( 'NONE', #482 ) ;
#14478=DIRECTION ( 'NONE',  ( -0.000000000000000000, -1.000000000000000000, -0.000000000000000000 ) ) ;
#14551=VERTEX_POINT ( 'NONE', #17188 ) ;
#14566=CARTESIAN_POINT ( 'NONE',  ( 0.000000000000000000, 0.4724409448818898127, 0.000000000000000000 ) ) ;
#14591=CARTESIAN_POINT ( 'NONE',  ( -1.692913385826771533, 0.07874015748031491790, -1.036610629921259805E-16 ) ) ;
#14593=AXIS2_PLACEMENT_3D ( 'NONE', #11305, #13291, #24294 ) ;
#14630=AXIS2_PLACEMENT_3D ( 'NONE', #11385, #13366, #17863 ) ;
#14648=DIRECTION ( 'NONE',  ( -0.000000000000000000, -1.000000000000000000, -0.000000000000000000 ) ) ;
#14674=CARTESIAN_POINT ( 'NONE',  ( -1.197070535079588716, 0.07874015748031495954, -1.197070535079588716 ) ) ;
#14698=ORIENTED_EDGE ( 'NONE', *, *, #20353, .T. ) ;
#14703=DIRECTION ( 'NONE',  ( 0.000000000000000000, -1.000000000000000000, 0.000000000000000000 ) ) ;
#14704=PLANE ( 'NONE',  #9148 ) ;
#14731=EDGE_LOOP ( 'NONE', ( #13978, #11837 ) ) ;
#14737=DIRECTION ( 'NONE',  ( 0.000000000000000000, -1.000000000000000000, 0.000000000000000000 ) ) ;
#14752=EDGE_LOOP ( 'NONE', ( #3981, #1991, #9967, #22091 ) ) ;
#14758=DIRECTION ( 'NONE',  ( 0.000000000000000000, 0.000000000000000000, 1.000000000000000000 ) ) ;
#14778=EDGE_CURVE ( 'NONE', #25308, #12497, #21228, .T. ) ;
#14813=CYLINDRICAL_SURFACE ( 'NONE', #4931, 0.1181102362204720091 ) ;
#14828=ORIENTED_EDGE ( 'NONE', *, *, #9051, .F. ) ;
#14838=CONICAL_SURFACE ( 'NONE', #23827, 0.2952755905511805778, 0.2617993875000016457 ) ;
#14857=EDGE_CURVE ( 'NONE', #27329, #21174, #19587, .T. ) ;
#14872=EDGE_CURVE ( 'NONE', #1498, #26351, #9645, .T. ) ;
#14876=ORIENTED_EDGE ( 'NONE', *, *, #24173, .T. ) ;
#14929=CARTESIAN_POINT ( 'NONE',  ( 9.642888182262624280E-17, 0.9055118110236221041, 0.7874015748031496509 ) ) ;
#14971=FACE_BOUND ( 'NONE', #11785, .T. ) ;
#14972=VERTEX_POINT ( 'NONE', #13423 ) ;
#14981=ORIENTED_EDGE ( 'NONE', *, *, #4333, .T. ) ;
#14990=EDGE_CURVE ( 'NONE', #9428, #7703, #26284, .T. ) ;
#15026=CIRCLE ( 'NONE', #19524, 0.1181102362204720091 ) ;
#15027=ORIENTED_EDGE ( 'NONE', *, *, #15197, .F. ) ;
#15032=DIRECTION ( 'NONE',  ( 0.000000000000000000, -1.000000000000000000, 0.000000000000000000 ) ) ;
#15050=ADVANCED_FACE ( 'NONE', ( #20349 ), #22605, .F. ) ;
#15053=ADVANCED_FACE ( 'NONE', ( #5376 ), #26840, .T. ) ;
#15078=CARTESIAN_POINT ( 'NONE',  ( 1.692913385826771533, 0.07874015748031495954, 0.1181102362204723144 ) ) ;
#15082=AXIS2_PLACEMENT_3D ( 'NONE', #8703, #17943, #11476 ) ;
#15137=FACE_OUTER_BOUND ( 'NONE', #24374, .T. ) ;
#15147=ADVANCED_FACE ( 'NONE', ( #1406 ), #5660, .F. ) ;
#15161=DIRECTION ( 'NONE',  ( 0.000000000000000000, 0.000000000000000000, -1.000000000000000000 ) ) ;
#15172=EDGE_LOOP ( 'NONE', ( #6344, #7465, #17237, #7832 ) ) ;
#15177=DIRECTION ( 'NONE',  ( -0.000000000000000000, -1.000000000000000000, -0.000000000000000000 ) ) ;
#15197=EDGE_CURVE ( 'NONE', #13490, #27656, #25478, .T. ) ;
#15218=CYLINDRICAL_SURFACE ( 'NONE', #15082, 0.1181102362204720091 ) ;
#15221=CIRCLE ( 'NONE', #16119, 1.988188976448617584 ) ;
#15262=DIRECTION ( 'NONE',  ( 0.000000000000000000, 0.000000000000000000, 1.000000000000000000 ) ) ;
#15271=EDGE_LOOP ( 'NONE', ( #24409, #4469 ) ) ;
#15306=ADVANCED_FACE ( 'NONE', ( #27833 ), #20504, .T. ) ;
#15310=ADVANCED_FACE ( 'NONE', ( #17228 ), #1552, .T. ) ;
#15312=ORIENTED_EDGE ( 'NONE', *, *, #12797, .T. ) ;
#15321=VERTEX_POINT ( 'NONE', #9272 ) ;
#15322=LINE ( 'NONE', #15583, #26563 ) ;
#15328=CARTESIAN_POINT ( 'NONE',  ( 0.000000000000000000, 0.07874015748031495954, 0.000000000000000000 ) ) ;
#15401=EDGE_CURVE ( 'NONE', #3555, #14474, #1553, .T. ) ;
#15409=AXIS2_PLACEMENT_3D ( 'NONE', #3899, #9832, #9691 ) ;
#15447=FACE_OUTER_BOUND ( 'NONE', #1776, .T. ) ;
#15477=DIRECTION ( 'NONE',  ( 0.000000000000000000, -1.000000000000000000, 0.000000000000000000 ) ) ;
#15508=AXIS2_PLACEMENT_3D ( 'NONE', #24527, #3043, #26374 ) ;
#15512=EDGE_LOOP ( 'NONE', ( #11084, #22781, #14346, #6796 ) ) ;
#15528=FACE_BOUND ( 'NONE', #3415, .T. ) ;
#15537=EDGE_CURVE ( 'NONE', #7099, #24215, #2186, .T. ) ;
#15557=CARTESIAN_POINT ( 'NONE',  ( 0.000000000000000000, 0.1968503937007875237, 0.000000000000000000 ) ) ;
#15571=CARTESIAN_POINT ( 'NONE',  ( 1.687505431895960050E-16, 0.4724409448818898127, -1.377952755905512472 ) ) ;
#15575=DIRECTION ( 'NONE',  ( 0.000000000000000000, 0.000000000000000000, -1.000000000000000000 ) ) ;
#15577=CARTESIAN_POINT ( 'NONE',  ( 9.642888182262624280E-17, 0.3543307086614173040, 0.7874015748031496509 ) ) ;
#15583=CARTESIAN_POINT ( 'NONE',  ( -1.692913385826771533, 0.07874015748031495954, -0.1181102362204721062 ) ) ;
#15590=ORIENTED_EDGE ( 'NONE', *, *, #27151, .T. ) ;
#15595=EDGE_CURVE ( 'NONE', #16430, #21688, #24569, .T. ) ;
#15603=CYLINDRICAL_SURFACE ( 'NONE', #25055, 1.377952755905512472 ) ;
#15619=CARTESIAN_POINT ( 'NONE',  ( -2.073220866141732523E-16, 0.07874015748031495954, 1.692913385826771533 ) ) ;
#15660=ADVANCED_FACE ( 'NONE', ( #11447 ), #24434, .F. ) ;
#15661=CIRCLE ( 'NONE', #26464, 1.988188976307287970 ) ;
#15668=EDGE_CURVE ( 'NONE', #16023, #25509, #8362, .T. ) ;
#15684=DIRECTION ( 'NONE',  ( 0.000000000000000000, -1.000000000000000000, 0.000000000000000000 ) ) ;
#15699=EDGE_CURVE ( 'NONE', #21158, #247, #5236, .T. ) ;
#15705=ORIENTED_EDGE ( 'NONE', *, *, #14778, .T. ) ;
#15723=ADVANCED_FACE ( 'NONE', ( #14442 ), #9899, .T. ) ;
#15756=CARTESIAN_POINT ( 'NONE',  ( 1.446433227339387294E-17, 0.07874015748031495954, -1.574803149606299524 ) ) ;
#15815=DIRECTION ( 'NONE',  ( 0.000000000000000000, -1.000000000000000000, 0.000000000000000000 ) ) ;
#15855=CIRCLE ( 'NONE', #5962, 0.1181102362204720091 ) ;
#15877=DIRECTION ( 'NONE',  ( -0.000000000000000000, -1.000000000000000000, -0.000000000000000000 ) ) ;
#15900=ORIENTED_EDGE ( 'NONE', *, *, #27381, .F. ) ;
#15909=DIRECTION ( 'NONE',  ( 0.000000000000000000, 0.000000000000000000, -1.000000000000000000 ) ) ;
#15934=VERTEX_POINT ( 'NONE', #17829 ) ;
#15967=DIRECTION ( 'NONE',  ( 0.000000000000000000, 0.000000000000000000, -1.000000000000000000 ) ) ;
#15975=( NAMED_UNIT ( * ) SI_UNIT ( $, .STERADIAN. ) SOLID_ANGLE_UNIT ( ) ) ;
#15982=EDGE_CURVE ( 'NONE', #21174, #7932, #2845, .T. ) ;
#15987=AXIS2_PLACEMENT_3D ( 'NONE', #6639, #2776, #15262 ) ;
#15991=AXIS2_PLACEMENT_3D ( 'NONE', #10430, #19045, #27679 ) ;
#16015=ORIENTED_EDGE ( 'NONE', *, *, #14275, .F. ) ;
#16023=VERTEX_POINT ( 'NONE', #12187 ) ;
#16039=VERTEX_POINT ( 'NONE', #23513 ) ;
#16048=EDGE_CURVE ( 'NONE', #13016, #9428, #9638, .T. ) ;
#16069=CARTESIAN_POINT ( 'NONE',  ( -1.197070535079588716, 0.07874015748031495954, 1.315180771300060503 ) ) ;
#16103=DIRECTION ( 'NONE',  ( 8.659560570126445370E-17, 0.7071067805519554161, -0.7071067818211396183 ) ) ;
#16116=EDGE_CURVE ( 'NONE', #7932, #8713, #27601, .T. ) ;
#16119=AXIS2_PLACEMENT_3D ( 'NONE', #10596, #19219, #10745 ) ;
#16145=DIRECTION ( 'NONE',  ( -0.000000000000000000, 1.000000000000000000, -0.000000000000000000 ) ) ;
#16165=DIRECTION ( 'NONE',  ( 0.000000000000000000, -1.000000000000000000, 0.000000000000000000 ) ) ;
#16173=DIRECTION ( 'NONE',  ( 0.000000000000000000, 0.000000000000000000, 1.000000000000000000 ) ) ;
#16197=VECTOR ( 'NONE', #3480, 39.37007874015748143 ) ;
#16243=CARTESIAN_POINT ( 'NONE',  ( 0.000000000000000000, 0.03937007874015747977, -0.3937007874015748254 ) ) ;
#16260=EDGE_LOOP ( 'NONE', ( #20414, #19061, #24901, #1662 ) ) ;
#16266=CARTESIAN_POINT ( 'NONE',  ( 0.000000000000000000, 0.07874015748031495954, 1.988188976307287970 ) ) ;
#16280=CARTESIAN_POINT ( 'NONE',  ( -1.197070535079588716, 0.4724409448818898127, 1.197070535079588716 ) ) ;
#16316=EDGE_LOOP ( 'NONE', ( #5292, #18444 ) ) ;
#16319=EDGE_CURVE ( 'NONE', #17190, #12564, #1353, .T. ) ;
#16335=DIRECTION ( 'NONE',  ( 0.000000000000000000, -1.000000000000000000, 0.000000000000000000 ) ) ;
#16348=CARTESIAN_POINT ( 'NONE',  ( 0.000000000000000000, 0.8661417322803149910, 0.000000000000000000 ) ) ;
#16356=CARTESIAN_POINT ( 'NONE',  ( 3.616083068348477634E-17, 0.000000000000000000, 0.2952755905511805778 ) ) ;
#16383=LINE ( 'NONE', #7914, #22278 ) ;
#16389=AXIS2_PLACEMENT_3D ( 'NONE', #8498, #200, #23762 ) ;
#16409=DIRECTION ( 'NONE',  ( 0.000000000000000000, -1.000000000000000000, 0.000000000000000000 ) ) ;
#16421=DIRECTION ( 'NONE',  ( -0.000000000000000000, -1.000000000000000000, -0.000000000000000000 ) ) ;
#16425=VERTEX_POINT ( 'NONE', #3672 ) ;
#16430=VERTEX_POINT ( 'NONE', #9900 ) ;
#16433=VECTOR ( 'NONE', #27442, 39.37007874015748143 ) ;
#16434=CARTESIAN_POINT ( 'NONE',  ( 0.000000000000000000, 0.07874015748031495954, 1.988188976307287970 ) ) ;
#16439=DIRECTION ( 'NONE',  ( 0.000000000000000000, 0.000000000000000000, -1.000000000000000000 ) ) ;
#16489=ORIENTED_EDGE ( 'NONE', *, *, #27381, .T. ) ;
#16491=EDGE_CURVE ( 'NONE', #16425, #19868, #20813, .T. ) ;
#16492=ORIENTED_EDGE ( 'NONE', *, *, #2812, .F. ) ;
#16518=DIRECTION ( 'NONE',  ( -0.000000000000000000, -1.000000000000000000, -0.000000000000000000 ) ) ;
#16519=CARTESIAN_POINT ( 'NONE',  ( 0.000000000000000000, 0.07874015748031508444, 0.000000000000000000 ) ) ;
#16521=EDGE_LOOP ( 'NONE', ( #7495, #19360, #8968, #5736 ) ) ;
#16523=ORIENTED_EDGE ( 'NONE', *, *, #16948, .F. ) ;
#16549=CIRCLE ( 'NONE', #5741, 0.1181102362204720091 ) ;
#16552=ORIENTED_EDGE ( 'NONE', *, *, #21093, .T. ) ;
#16562=DIRECTION ( 'NONE',  ( 0.000000000000000000, 0.000000000000000000, -1.000000000000000000 ) ) ;
#16564=VERTEX_POINT ( 'NONE', #23484 ) ;
#16592=ORIENTED_EDGE ( 'NONE', *, *, #15699, .F. ) ;
#16595=SHAPE_DEFINITION_REPRESENTATION ( #5079, #4612 ) ;
#16611=DIRECTION ( 'NONE',  ( 0.000000000000000000, 0.000000000000000000, -1.000000000000000000 ) ) ;
#16653=FACE_BOUND ( 'NONE', #20225, .T. ) ;
#16735=CARTESIAN_POINT ( 'NONE',  ( 3.616083068348477634E-17, 0.07874015748662489822, 0.2952755905511805778 ) ) ;
#16825=ORIENTED_EDGE ( 'NONE', *, *, #17689, .F. ) ;
#16858=EDGE_CURVE ( 'NONE', #16039, #16425, #21131, .T. ) ;
#16873=CYLINDRICAL_SURFACE ( 'NONE', #21742, 0.7874015748031496509 ) ;
#16896=DIRECTION ( 'NONE',  ( 0.000000000000000000, -1.000000000000000000, 0.000000000000000000 ) ) ;
#16941=EDGE_LOOP ( 'NONE', ( #27145, #25503, #20106, #16592 ) ) ;
#16948=EDGE_CURVE ( 'NONE', #12564, #23913, #1331, .T. ) ;
#16951=VECTOR ( 'NONE', #755, 39.37007874015748143 ) ;
#16958=DIRECTION ( 'NONE',  ( 3.169619147893061878E-17, -0.9659258263664941557, 0.2588190448135637145 ) ) ;
#16959=EDGE_LOOP ( 'NONE', ( #7555, #17987, #17858, #27674 ) ) ;
#16968=ORIENTED_EDGE ( 'NONE', *, *, #10642, .T. ) ;
#16993=ORIENTED_EDGE ( 'NONE', *, *, #14857, .T. ) ;
#16997=DIRECTION ( 'NONE',  ( 0.000000000000000000, -1.000000000000000000, 0.000000000000000000 ) ) ;
#16998=DIRECTION ( 'NONE',  ( 0.000000000000000000, 0.000000000000000000, -1.000000000000000000 ) ) ;
#17046=LINE ( 'NONE', #27364, #19156 ) ;
#17076=ORIENTED_EDGE ( 'NONE', *, *, #8160, .F. ) ;
#17087=CIRCLE ( 'NONE', #12116, 0.1181102362204718703 ) ;
#17091=CARTESIAN_POINT ( 'NONE',  ( 0.000000000000000000, 0.5905511811023621549, 0.000000000000000000 ) ) ;
#17120=DIRECTION ( 'NONE',  ( 0.000000000000000000, 0.000000000000000000, -1.000000000000000000 ) ) ;
#17126=CONICAL_SURFACE ( 'NONE', #4504, 0.5511811023975373702, 0.7853981633974482790 ) ;
#17133=FACE_BOUND ( 'NONE', #13481, .T. ) ;
#17145=FACE_OUTER_BOUND ( 'NONE', #27037, .T. ) ;
#17147=DIRECTION ( 'NONE',  ( 0.000000000000000000, 1.000000000000000000, 0.000000000000000000 ) ) ;
#17157=EDGE_LOOP ( 'NONE', ( #26021, #13829, #2689, #1790 ) ) ;
#17168=ORIENTED_EDGE ( 'NONE', *, *, #26852, .T. ) ;
#17170=ORIENTED_EDGE ( 'NONE', *, *, #9171, .T. ) ;
#17182=DIRECTION ( 'NONE',  ( -0.000000000000000000, -1.000000000000000000, -0.000000000000000000 ) ) ;
#17188=CARTESIAN_POINT ( 'NONE',  ( 6.991093932464927839E-17, 0.03937007874015751446, -0.5511811023975373702 ) ) ;
#17190=VERTEX_POINT ( 'NONE', #27319 ) ;
#17191=CARTESIAN_POINT ( 'NONE',  ( -1.197070535079588716, 0.07874015748031495954, -1.078960298859116707 ) ) ;
#17205=ORIENTED_EDGE ( 'NONE', *, *, #18848, .F. ) ;
#17214=DIRECTION ( 'NONE',  ( 0.000000000000000000, 0.000000000000000000, -1.000000000000000000 ) ) ;
#17228=FACE_OUTER_BOUND ( 'NONE', #14431, .T. ) ;
#17237=ORIENTED_EDGE ( 'NONE', *, *, #5885, .T. ) ;
#17239=CARTESIAN_POINT ( 'NONE',  ( 0.000000000000000000, 0.3937007873309092409, 0.000000000000000000 ) ) ;
#17264=CARTESIAN_POINT ( 'NONE',  ( 4.821444091131312140E-17, 0.1968503937007874127, 0.3937007874015748254 ) ) ;
#17266=CIRCLE ( 'NONE', #1027, 1.377952755905512472 ) ;
#17290=CARTESIAN_POINT ( 'NONE',  ( -1.197070535079588716, 0.4724409448818898127, 1.197070535079588716 ) ) ;
#17295=ORIENTED_EDGE ( 'NONE', *, *, #9482, .F. ) ;
#17298=DIRECTION ( 'NONE',  ( 0.000000000000000000, -1.000000000000000000, 0.000000000000000000 ) ) ;
#17313=FACE_BOUND ( 'NONE', #4880, .T. ) ;
#17325=AXIS2_PLACEMENT_3D ( 'NONE', #6673, #17796, #9310 ) ;
#17381=VERTEX_POINT ( 'NONE', #24314 ) ;
#17391=VECTOR ( 'NONE', #10465, 39.37007874015748143 ) ;
#17468=FACE_OUTER_BOUND ( 'NONE', #2550, .T. ) ;
#17486=COLOUR_RGB ( '', 0.09019608, 0.27058824, 0.51372549) ;
#17502=VERTEX_POINT ( 'NONE', #27424 ) ;
#17521=CARTESIAN_POINT ( 'NONE',  ( 9.642888182478974314E-17, 0.1968503937007874127, 0.7874015748208159637 ) ) ;
#17533=CARTESIAN_POINT ( 'NONE',  ( 0.000000000000000000, 0.4724409448818898127, 0.000000000000000000 ) ) ;
#17535=CONICAL_SURFACE ( 'NONE', #13034, 2.066929133858267598, 0.7853981624999996081 ) ;
#17537=VERTEX_POINT ( 'NONE', #19365 ) ;
#17547=FACE_BOUND ( 'NONE', #11595, .T. ) ;
#17549=EDGE_LOOP ( 'NONE', ( #4141, #7750 ) ) ;
#17557=LINE ( 'NONE', #21384, #9093 ) ;
#17560=DIRECTION ( 'NONE',  ( 0.000000000000000000, 0.000000000000000000, 1.000000000000000000 ) ) ;
#17571=VECTOR ( 'NONE', #19685, 39.37007874015748854 ) ;
#17607=ADVANCED_FACE ( 'NONE', ( #21490 ), #24017, .T. ) ;
#17610=DIRECTION ( 'NONE',  ( 0.000000000000000000, 0.000000000000000000, -1.000000000000000000 ) ) ;
#17633=CIRCLE ( 'NONE', #15409, 0.1181102362204720091 ) ;
#17644=ORIENTED_EDGE ( 'NONE', *, *, #24503, .F. ) ;
#17668=CYLINDRICAL_SURFACE ( 'NONE', #27331, 0.3937007874015748254 ) ;
#17670=FACE_BOUND ( 'NONE', #24653, .T. ) ;
#17689=EDGE_CURVE ( 'NONE', #12475, #14000, #26072, .T. ) ;
#17691=EDGE_CURVE ( 'NONE', #24515, #23576, #12094, .T. ) ;
#17708=DIRECTION ( 'NONE',  ( -0.000000000000000000, 1.000000000000000000, -0.000000000000000000 ) ) ;
#17709=DIRECTION ( 'NONE',  ( 0.000000000000000000, 0.000000000000000000, -1.000000000000000000 ) ) ;
#17724=VERTEX_POINT ( 'NONE', #16243 ) ;
#17734=ORIENTED_EDGE ( 'NONE', *, *, #23952, .F. ) ;
#17796=DIRECTION ( 'NONE',  ( -0.000000000000000000, -1.000000000000000000, -0.000000000000000000 ) ) ;
#17806=AXIS2_PLACEMENT_3D ( 'NONE', #14394, #23005, #24824 ) ;
#17829=CARTESIAN_POINT ( 'NONE',  ( 0.000000000000000000, 0.07874015746264864668, -0.7874015748208159637 ) ) ;
#17842=ORIENTED_EDGE ( 'NONE', *, *, #27668, .F. ) ;
#17858=ORIENTED_EDGE ( 'NONE', *, *, #9482, .T. ) ;
#17863=DIRECTION ( 'NONE',  ( 0.000000000000000000, 0.000000000000000000, -1.000000000000000000 ) ) ;
#17864=ORIENTED_EDGE ( 'NONE', *, *, #16491, .F. ) ;
#17905=CARTESIAN_POINT ( 'NONE',  ( 2.531258147843938596E-16, 0.4724409448818898127, 2.066929133858267598 ) ) ;
#17917=CARTESIAN_POINT ( 'NONE',  ( 1.197070535079588716, 0.07874015748031495954, -1.197070535079588716 ) ) ;
#17924=FACE_OUTER_BOUND ( 'NONE', #24879, .T. ) ;
#17928=ORIENTED_EDGE ( 'NONE', *, *, #19361, .F. ) ;
#17943=DIRECTION ( 'NONE',  ( -0.000000000000000000, -1.000000000000000000, -0.000000000000000000 ) ) ;
#17956=DIRECTION ( 'NONE',  ( -0.000000000000000000, 1.000000000000000000, 0.000000000000000000 ) ) ;
#17970=CARTESIAN_POINT ( 'NONE',  ( 0.000000000000000000, 0.9055118110236221041, -0.7874015748031496509 ) ) ;
#17987=ORIENTED_EDGE ( 'NONE', *, *, #3120, .T. ) ;
#17993=ORIENTED_EDGE ( 'NONE', *, *, #26276, .T. ) ;
#18047=CARTESIAN_POINT ( 'NONE',  ( 0.000000000000000000, 0.07874015748031508444, -1.377952755905512472 ) ) ;
#18103=CARTESIAN_POINT ( 'NONE',  ( 0.000000000000000000, 0.8661417322803149910, -0.3937007874015748254 ) ) ;
#18109=ORIENTED_EDGE ( 'NONE', *, *, #3685, .F. ) ;
#18126=ORIENTED_EDGE ( 'NONE', *, *, #10071, .F. ) ;
#18129=EDGE_LOOP ( 'NONE', ( #26834, #9618 ) ) ;
#18201=DIRECTION ( 'NONE',  ( 0.000000000000000000, 0.000000000000000000, 1.000000000000000000 ) ) ;
#18204=CIRCLE ( 'NONE', #2878, 0.7874015748208159637 ) ;
#18205=( NAMED_UNIT ( * ) PLANE_ANGLE_UNIT ( ) SI_UNIT ( $, .RADIAN. ) ) ;
#18219=AXIS2_PLACEMENT_3D ( 'NONE', #17091, #23332, #3956 ) ;
#18244=CIRCLE ( 'NONE', #5171, 1.377952755905512472 ) ;
#18245=FACE_BOUND ( 'NONE', #5666, .T. ) ;
#18249=ORIENTED_EDGE ( 'NONE', *, *, #5314, .F. ) ;
#18251=DIRECTION ( 'NONE',  ( 0.000000000000000000, 0.000000000000000000, -1.000000000000000000 ) ) ;
#18257=FACE_OUTER_BOUND ( 'NONE', #493, .T. ) ;
#18270=DIRECTION ( 'NONE',  ( -0.000000000000000000, 1.000000000000000000, -0.000000000000000000 ) ) ;
#18301=VERTEX_POINT ( 'NONE', #5756 ) ;
#18389=CARTESIAN_POINT ( 'NONE',  ( 0.000000000000000000, 0.03937007874015747977, 0.000000000000000000 ) ) ;
#18405=ORIENTED_EDGE ( 'NONE', *, *, #13013, .T. ) ;
#18413=AXIS2_PLACEMENT_3D ( 'NONE', #436, #16335, #5459 ) ;
#18425=CYLINDRICAL_SURFACE ( 'NONE', #18413, 2.066929133858267598 ) ;
#18444=ORIENTED_EDGE ( 'NONE', *, *, #33, .F. ) ;
#18474=DIRECTION ( 'NONE',  ( 0.000000000000000000, 0.000000000000000000, -1.000000000000000000 ) ) ;
#18477=AXIS2_PLACEMENT_3D ( 'NONE', #14591, #3525, #12152 ) ;
#18523=EDGE_CURVE ( 'NONE', #10848, #7459, #13470, .T. ) ;
#18525=VECTOR ( 'NONE', #19577, 39.37007874015748143 ) ;
#18565=DIRECTION ( 'NONE',  ( 0.000000000000000000, 0.000000000000000000, -1.000000000000000000 ) ) ;
#18608=ORIENTED_EDGE ( 'NONE', *, *, #16491, .T. ) ;
#18617=DIRECTION ( 'NONE',  ( -0.000000000000000000, 1.000000000000000000, -0.000000000000000000 ) ) ;
#18630=ORIENTED_EDGE ( 'NONE', *, *, #22166, .T. ) ;
#18639=CARTESIAN_POINT ( 'NONE',  ( 1.692913385826771533, 0.07874015748031491790, 0.1181102362204723144 ) ) ;
#18658=AXIS2_PLACEMENT_3D ( 'NONE', #12885, #15032, #19389 ) ;
#18674=CARTESIAN_POINT ( 'NONE',  ( 0.000000000000000000, 0.9055118110236217710, -0.2952755905511805223 ) ) ;
#18715=DIRECTION ( 'NONE',  ( -0.000000000000000000, -1.000000000000000000, -0.000000000000000000 ) ) ;
#18721=ORIENTED_EDGE ( 'NONE', *, *, #5252, .F. ) ;
#18728=DIRECTION ( 'NONE',  ( 0.000000000000000000, -1.000000000000000000, 0.000000000000000000 ) ) ;
#18733=CARTESIAN_POINT ( 'NONE',  ( 1.197070535079588716, 0.07874015748031491790, -1.197070535079588716 ) ) ;
#18780=( CONVERSION_BASED_UNIT ( 'INCH', #3095 ) LENGTH_UNIT ( ) NAMED_UNIT ( #2933 ) ) ;
#18783=CIRCLE ( 'NONE', #11133, 0.4921259842519685179 ) ;
#18787=ORIENTED_EDGE ( 'NONE', *, *, #19106, .T. ) ;
#18819=EDGE_LOOP ( 'NONE', ( #9999, #24043 ) ) ;
#18837=AXIS2_PLACEMENT_3D ( 'NONE', #11536, #20152, #14200 ) ;
#18848=EDGE_CURVE ( 'NONE', #17724, #25308, #4812, .T. ) ;
#18866=DIRECTION ( 'NONE',  ( -0.000000000000000000, -1.000000000000000000, -0.000000000000000000 ) ) ;
#18867=DIRECTION ( 'NONE',  ( 0.000000000000000000, -1.000000000000000000, 0.000000000000000000 ) ) ;
#18894=AXIS2_PLACEMENT_3D ( 'NONE', #4454, #24080, #2460 ) ;
#18901=DIRECTION ( 'NONE',  ( 0.000000000000000000, -1.000000000000000000, 0.000000000000000000 ) ) ;
#18915=DIRECTION ( 'NONE',  ( 0.000000000000000000, 0.000000000000000000, -1.000000000000000000 ) ) ;
#18919=DIMENSIONAL_EXPONENTS ( 1.000000000000000000, 0.000000000000000000, 0.000000000000000000, 0.000000000000000000, 0.000000000000000000, 0.000000000000000000, 0.000000000000000000 ) ;
#18930=CARTESIAN_POINT ( 'NONE',  ( 0.000000000000000000, 0.9055118110236221041, -0.4921259842519685179 ) ) ;
#18936=ORIENTED_EDGE ( 'NONE', *, *, #27793, .T. ) ;
#18971=CARTESIAN_POINT ( 'NONE',  ( 0.000000000000000000, 0.9055118110236221041, 0.000000000000000000 ) ) ;
#18986=VERTEX_POINT ( 'NONE', #3471 ) ;
#19001=EDGE_LOOP ( 'NONE', ( #18630, #11344, #21839, #12054 ) ) ;
#19027=ORIENTED_EDGE ( 'NONE', *, *, #15401, .F. ) ;
#19045=DIRECTION ( 'NONE',  ( -0.000000000000000000, -1.000000000000000000, -0.000000000000000000 ) ) ;
#19061=ORIENTED_EDGE ( 'NONE', *, *, #14990, .T. ) ;
#19078=DIRECTION ( 'NONE',  ( 0.000000000000000000, -1.000000000000000000, 0.000000000000000000 ) ) ;
#19106=EDGE_CURVE ( 'NONE', #19868, #16425, #12925, .T. ) ;
#19156=VECTOR ( 'NONE', #20856, 39.37007874015748143 ) ;
#19157=CARTESIAN_POINT ( 'NONE',  ( 0.000000000000000000, 0.3543307086614173040, -0.7874015748031496509 ) ) ;
#19182=VECTOR ( 'NONE', #17298, 39.37007874015748143 ) ;
#19201=AXIS2_PLACEMENT_3D ( 'NONE', #22189, #26697, #726 ) ;
#19206=CIRCLE ( 'NONE', #5221, 0.1181102362204718703 ) ;
#19219=DIRECTION ( 'NONE',  ( -0.000000000000000000, 1.000000000000000000, -0.000000000000000000 ) ) ;
#19224=CARTESIAN_POINT ( 'NONE',  ( 0.000000000000000000, 0.07874015748031495954, -1.811023622047243542 ) ) ;
#19230=CARTESIAN_POINT ( 'NONE',  ( 0.000000000000000000, 0.03937007874015751446, 0.000000000000000000 ) ) ;
#19237=ORIENTED_EDGE ( 'NONE', *, *, #11979, .F. ) ;
#19249=FACE_BOUND ( 'NONE', #9184, .T. ) ;
#19255=DIRECTION ( 'NONE',  ( 0.000000000000000000, 0.000000000000000000, 1.000000000000000000 ) ) ;
#19295=FACE_OUTER_BOUND ( 'NONE', #5420, .T. ) ;
#19306=FACE_OUTER_BOUND ( 'NONE', #26683, .T. ) ;
#19320=VERTEX_POINT ( 'NONE', #2835 ) ;
#19328=EDGE_CURVE ( 'NONE', #7057, #21158, #15661, .T. ) ;
#19360=ORIENTED_EDGE ( 'NONE', *, *, #25196, .T. ) ;
#19361=EDGE_CURVE ( 'NONE', #14467, #17381, #19206, .T. ) ;
#19365=CARTESIAN_POINT ( 'NONE',  ( -1.197070535079588716, 0.07874015748031491790, -1.315180771300060503 ) ) ;
#19370=CARTESIAN_POINT ( 'NONE',  ( -1.928577543407793639E-16, 0.07874015748031495954, 1.811023622047243542 ) ) ;
#19389=DIRECTION ( 'NONE',  ( 0.000000000000000000, -0.000000000000000000, -1.000000000000000000 ) ) ;
#19435=CARTESIAN_POINT ( 'NONE',  ( 0.3937007874015748254, 0.03937007874015750059, 0.000000000000000000 ) ) ;
#19458=VERTEX_POINT ( 'NONE', #5593 ) ;
#19459=ORIENTED_EDGE ( 'NONE', *, *, #9171, .F. ) ;
#19478=EDGE_CURVE ( 'NONE', #19320, #1582, #1616, .T. ) ;
#19500=CARTESIAN_POINT ( 'NONE',  ( 0.000000000000000000, 0.4724409448818898127, 0.000000000000000000 ) ) ;
#19513=DIRECTION ( 'NONE',  ( -0.000000000000000000, 1.000000000000000000, -0.000000000000000000 ) ) ;
#19524=AXIS2_PLACEMENT_3D ( 'NONE', #7475, #7067, #9296 ) ;
#19577=DIRECTION ( 'NONE',  ( -0.000000000000000000, -1.000000000000000000, -0.000000000000000000 ) ) ;
#19587=CIRCLE ( 'NONE', #12360, 0.2952755905511805223 ) ;
#19640=DIRECTION ( 'NONE',  ( -0.000000000000000000, -1.000000000000000000, -0.000000000000000000 ) ) ;
#19662=CARTESIAN_POINT ( 'NONE',  ( 0.000000000000000000, 0.4724409448818898127, -0.7874015748031496509 ) ) ;
#19666=ORIENTED_EDGE ( 'NONE', *, *, #10264, .F. ) ;
#19678=AXIS2_PLACEMENT_3D ( 'NONE', #20139, #3168, #24792 ) ;
#19682=DIRECTION ( 'NONE',  ( -0.000000000000000000, 1.000000000000000000, -0.000000000000000000 ) ) ;
#19685=DIRECTION ( 'NONE',  ( 8.659560562354932858E-17, 0.7071067811865474617, -0.7071067811865474617 ) ) ;
#19701=CARTESIAN_POINT ( 'NONE',  ( 1.692913385826771533, 0.07874015748031495954, 3.109831496062992451E-16 ) ) ;
#19709=CIRCLE ( 'NONE', #12923, 0.1181102362204718703 ) ;
#19762=CIRCLE ( 'NONE', #22462, 0.1181102362204718703 ) ;
#19783=AXIS2_PLACEMENT_3D ( 'NONE', #25735, #201, #17120 ) ;
#19811=CARTESIAN_POINT ( 'NONE',  ( 6.750021728016536817E-17, 0.03937007874015751446, -0.5511811023975373702 ) ) ;
#19813=DIRECTION ( 'NONE',  ( 0.000000000000000000, 0.000000000000000000, -1.000000000000000000 ) ) ;
#19823=DIRECTION ( 'NONE',  ( -0.000000000000000000, 1.000000000000000000, -0.000000000000000000 ) ) ;
#19843=CARTESIAN_POINT ( 'NONE',  ( 1.197070535079588716, 0.4724409448818898127, 1.197070535079588716 ) ) ;
#19864=ADVANCED_FACE ( 'NONE', ( #9214, #18245 ), #759, .T. ) ;
#19868=VERTEX_POINT ( 'NONE', #11620 ) ;
#19920=AXIS2_PLACEMENT_3D ( 'NONE', #15557, #4789, #13408 ) ;
#19922=DIRECTION ( 'NONE',  ( 0.000000000000000000, -0.000000000000000000, -1.000000000000000000 ) ) ;
#19927=CARTESIAN_POINT ( 'NONE',  ( 0.5905511811200284678, 0.07874015746264864668, 0.000000000000000000 ) ) ;
#19993=EDGE_CURVE ( 'NONE', #14972, #20570, #6616, .T. ) ;
#20012=CIRCLE ( 'NONE', #8294, 0.1181102362204718703 ) ;
#20020=DIRECTION ( 'NONE',  ( 0.000000000000000000, -0.000000000000000000, -1.000000000000000000 ) ) ;
#20042=CARTESIAN_POINT ( 'NONE',  ( 1.197070535079588716, 0.07874015748031495954, 1.197070535079588716 ) ) ;
#20050=DIRECTION ( 'NONE',  ( 0.000000000000000000, 0.000000000000000000, 1.000000000000000000 ) ) ;
#20055=DIRECTION ( 'NONE',  ( 0.000000000000000000, 0.000000000000000000, 1.000000000000000000 ) ) ;
#20088=CARTESIAN_POINT ( 'NONE',  ( 0.000000000000000000, 0.07874015748031495954, 0.000000000000000000 ) ) ;
#20106=ORIENTED_EDGE ( 'NONE', *, *, #7382, .F. ) ;
#20139=CARTESIAN_POINT ( 'NONE',  ( 0.000000000000000000, 0.07874015746264864668, 0.000000000000000000 ) ) ;
#20146=ORIENTED_EDGE ( 'NONE', *, *, #22485, .F. ) ;
#20152=DIRECTION ( 'NONE',  ( 0.000000000000000000, -1.000000000000000000, 0.000000000000000000 ) ) ;
#20162=CARTESIAN_POINT ( 'NONE',  ( 0.000000000000000000, 0.1574803148899641958, -2.066929133858267598 ) ) ;
#20184=CIRCLE ( 'NONE', #8028, 0.1181102362204720091 ) ;
#20192=FACE_OUTER_BOUND ( 'NONE', #11260, .T. ) ;
#20200=AXIS2_PLACEMENT_3D ( 'NONE', #11637, #26748, #7544 ) ;
#20203=DIRECTION ( 'NONE',  ( -0.000000000000000000, 1.000000000000000000, -0.000000000000000000 ) ) ;
#20205=AXIS2_PLACEMENT_3D ( 'NONE', #8077, #19078, #12449 ) ;
#20225=EDGE_LOOP ( 'NONE', ( #2122, #9721 ) ) ;
#20244=DIRECTION ( 'NONE',  ( 0.000000000000000000, 0.000000000000000000, 1.000000000000000000 ) ) ;
#20301=PLANE ( 'NONE',  #22709 ) ;
#20332=CARTESIAN_POINT ( 'NONE',  ( 0.000000000000000000, -1.533249767903113305E-16, 0.000000000000000000 ) ) ;
#20349=FACE_OUTER_BOUND ( 'NONE', #16260, .T. ) ;
#20351=DIRECTION ( 'NONE',  ( 0.000000000000000000, -1.000000000000000000, 0.000000000000000000 ) ) ;
#20353=EDGE_CURVE ( 'NONE', #372, #17537, #26698, .T. ) ;
#20392=CARTESIAN_POINT ( 'NONE',  ( 0.000000000000000000, 0.1968503937007874127, -0.7874015748208159637 ) ) ;
#20393=CARTESIAN_POINT ( 'NONE',  ( 0.000000000000000000, -1.707404996040164512E-16, 0.000000000000000000 ) ) ;
#20414=ORIENTED_EDGE ( 'NONE', *, *, #11461, .F. ) ;
#20456=CARTESIAN_POINT ( 'NONE',  ( 0.000000000000000000, 0.4724409448818896462, 1.377952755905512472 ) ) ;
#20475=CARTESIAN_POINT ( 'NONE',  ( 1.197070535079588716, 0.07874015748031491790, 1.197070535079588716 ) ) ;
#20490=CIRCLE ( 'NONE', #21844, 0.7874015748208159637 ) ;
#20492=ORIENTED_EDGE ( 'NONE', *, *, #8372, .T. ) ;
#20504=CONICAL_SURFACE ( 'NONE', #11465, 0.3937007874015748254, 0.2617993874999990922 ) ;
#20510=ORIENTED_EDGE ( 'NONE', *, *, #26212, .F. ) ;
#20522=ORIENTED_EDGE ( 'NONE', *, *, #27592, .F. ) ;
#20545=DIRECTION ( 'NONE',  ( -0.000000000000000000, 1.000000000000000000, -0.000000000000000000 ) ) ;
#20570=VERTEX_POINT ( 'NONE', #27142 ) ;
#20571=EDGE_CURVE ( 'NONE', #20570, #14972, #25642, .T. ) ;
#20583=CARTESIAN_POINT ( 'NONE',  ( 0.000000000000000000, 0.1968503937007874127, 0.000000000000000000 ) ) ;
#20625=DIRECTION ( 'NONE',  ( -0.000000000000000000, -1.000000000000000000, -0.000000000000000000 ) ) ;
#20645=CARTESIAN_POINT ( 'NONE',  ( 1.197070535079588716, 0.07874015748031495954, -1.197070535079588716 ) ) ;
#20732=AXIS2_PLACEMENT_3D ( 'NONE', #19435, #18867, #10536 ) ;
#20738=ADVANCED_FACE ( 'NONE', ( #15137 ), #17535, .T. ) ;
#20752=EDGE_CURVE ( 'NONE', #18986, #18301, #865, .T. ) ;
#20764=ADVANCED_FACE ( 'NONE', ( #22408 ), #18425, .T. ) ;
#20811=CARTESIAN_POINT ( 'NONE',  ( 6.026805113914139867E-17, 0.5905511811023621549, 0.4921259842519685179 ) ) ;
#20813=CIRCLE ( 'NONE', #18477, 0.1181102362204720091 ) ;
#20836=EDGE_CURVE ( 'NONE', #22837, #15321, #12788, .T. ) ;
#20856=DIRECTION ( 'NONE',  ( 0.000000000000000000, -1.000000000000000000, 0.000000000000000000 ) ) ;
#20918=AXIS2_PLACEMENT_3D ( 'NONE', #9441, #9302, #19922 ) ;
#20923=ADVANCED_FACE ( 'NONE', ( #21547 ), #10810, .F. ) ;
#20948=ORIENTED_EDGE ( 'NONE', *, *, #27506, .T. ) ;
#20985=ORIENTED_EDGE ( 'NONE', *, *, #2973, .T. ) ;
#21093=EDGE_CURVE ( 'NONE', #20570, #15934, #11774, .T. ) ;
#21112=CONICAL_SURFACE ( 'NONE', #27050, 1.988188976307287970, 0.7853981642948970610 ) ;
#21119=ORIENTED_EDGE ( 'NONE', *, *, #5252, .T. ) ;
#21130=CYLINDRICAL_SURFACE ( 'NONE', #4547, 0.1181102362204718703 ) ;
#21131=LINE ( 'NONE', #10386, #23021 ) ;
#21158=VERTEX_POINT ( 'NONE', #16434 ) ;
#21161=AXIS2_PLACEMENT_3D ( 'NONE', #19927, #1000, #9449 ) ;
#21174=VERTEX_POINT ( 'NONE', #18674 ) ;
#21219=FACE_OUTER_BOUND ( 'NONE', #17157, .T. ) ;
#21222=VECTOR ( 'NONE', #15815, 39.37007874015748143 ) ;
#21228=LINE ( 'NONE', #17264, #16433 ) ;
#21245=DIRECTION ( 'NONE',  ( -0.000000000000000000, -1.000000000000000000, -0.000000000000000000 ) ) ;
#21260=ORIENTED_EDGE ( 'NONE', *, *, #5680, .T. ) ;
#21262=CARTESIAN_POINT ( 'NONE',  ( 4.821444091131312140E-17, -1.707404996040164512E-16, 0.3937007874015748254 ) ) ;
#21289=EDGE_CURVE ( 'NONE', #9880, #19868, #15322, .T. ) ;
#21293=EDGE_LOOP ( 'NONE', ( #6023, #25461, #10965, #16015 ) ) ;
#21295=ORIENTED_EDGE ( 'NONE', *, *, #7766, .T. ) ;
#21300=EDGE_LOOP ( 'NONE', ( #7608, #22296 ) ) ;
#21310=ORIENTED_EDGE ( 'NONE', *, *, #27151, .F. ) ;
#21384=CARTESIAN_POINT ( 'NONE',  ( 1.197070535079588716, 0.07874015748031495954, -1.315180771300060503 ) ) ;
#21386=EDGE_LOOP ( 'NONE', ( #7796, #22664 ) ) ;
#21395=CARTESIAN_POINT ( 'NONE',  ( 0.000000000000000000, 0.8661417322803149910, -0.3937007874015748254 ) ) ;
#21430=ORIENTED_EDGE ( 'NONE', *, *, #1826, .F. ) ;
#21441=EDGE_CURVE ( 'NONE', #14551, #11993, #27435, .T. ) ;
#21454=AXIS2_PLACEMENT_3D ( 'NONE', #17917, #13149, #21502 ) ;
#21490=FACE_OUTER_BOUND ( 'NONE', #8507, .T. ) ;
#21494=AXIS2_PLACEMENT_3D ( 'NONE', #7817, #16997, #10195 ) ;
#21502=DIRECTION ( 'NONE',  ( 0.000000000000000000, 0.000000000000000000, -1.000000000000000000 ) ) ;
#21547=FACE_OUTER_BOUND ( 'NONE', #15172, .T. ) ;
#21553=SURFACE_STYLE_USAGE ( .BOTH. , #384 ) ;
#21588=CARTESIAN_POINT ( 'NONE',  ( -1.928577543407793639E-16, 0.07874015748031491790, 1.811023622047243542 ) ) ;
#21617=ORIENTED_EDGE ( 'NONE', *, *, #24672, .F. ) ;
#21688=VERTEX_POINT ( 'NONE', #24155 ) ;
#21691=AXIS2_PLACEMENT_3D ( 'NONE', #3749, #27211, #25082 ) ;
#21696=CARTESIAN_POINT ( 'NONE',  ( 1.687505431895960050E-16, 0.4724409448818896462, -1.377952755905512472 ) ) ;
#21714=CARTESIAN_POINT ( 'NONE',  ( -1.692913385826771533, 0.07874015748031495954, -1.036610629921259805E-16 ) ) ;
#21742=AXIS2_PLACEMENT_3D ( 'NONE', #18971, #12193, #16439 ) ;
#21782=ADVANCED_FACE ( 'NONE', ( #17468 ), #26082, .F. ) ;
#21783=CIRCLE ( 'NONE', #1939, 0.1181102362204718703 ) ;
#21825=AXIS2_PLACEMENT_3D ( 'NONE', #14248, #3478, #12391 ) ;
#21828=CARTESIAN_POINT ( 'NONE',  ( 3.616083068348477018E-17, 0.9055118110236217710, 0.2952755905511805223 ) ) ;
#21831=DIRECTION ( 'NONE',  ( -0.000000000000000000, -1.000000000000000000, -0.000000000000000000 ) ) ;
#21839=ORIENTED_EDGE ( 'NONE', *, *, #24019, .T. ) ;
#21844=AXIS2_PLACEMENT_3D ( 'NONE', #23373, #6136, #16562 ) ;
#21860=ORIENTED_EDGE ( 'NONE', *, *, #3257, .T. ) ;
#21866=EDGE_LOOP ( 'NONE', ( #27064, #15312, #9388, #10664 ) ) ;
#21877=AXIS2_PLACEMENT_3D ( 'NONE', #6053, #12537, #10688 ) ;
#21973=CARTESIAN_POINT ( 'NONE',  ( 0.000000000000000000, 0.03937007874015751446, 0.000000000000000000 ) ) ;
#21986=ORIENTED_EDGE ( 'NONE', *, *, #8529, .F. ) ;
#22025=CARTESIAN_POINT ( 'NONE',  ( 0.000000000000000000, 0.3937007873309092409, 0.000000000000000000 ) ) ;
#22086=ORIENTED_EDGE ( 'NONE', *, *, #12519, .F. ) ;
#22091=ORIENTED_EDGE ( 'NONE', *, *, #7586, .T. ) ;
#22132=ORIENTED_EDGE ( 'NONE', *, *, #26276, .F. ) ;
#22139=FACE_OUTER_BOUND ( 'NONE', #3960, .T. ) ;
#22153=ORIENTED_EDGE ( 'NONE', *, *, #8214, .T. ) ;
#22166=EDGE_CURVE ( 'NONE', #12080, #13707, #20184, .T. ) ;
#22178=EDGE_LOOP ( 'NONE', ( #1089, #18249, #24401, #25345 ) ) ;
#22182=PLANE ( 'NONE',  #21161 ) ;
#22189=CARTESIAN_POINT ( 'NONE',  ( 0.000000000000000000, 0.9055118110236221041, 0.000000000000000000 ) ) ;
#22231=VECTOR ( 'NONE', #26607, 39.37007874015748143 ) ;
#22233=CARTESIAN_POINT ( 'NONE',  ( 1.692913385826771533, 0.07874015748031495954, -0.1181102362204716899 ) ) ;
#22247=AXIS2_PLACEMENT_3D ( 'NONE', #4560, #353, #17560 ) ;
#22261=ORIENTED_EDGE ( 'NONE', *, *, #15982, .F. ) ;
#22278=VECTOR ( 'NONE', #5799, 39.37007874015748854 ) ;
#22286=CONICAL_SURFACE ( 'NONE', #12818, 0.3937007874015748254, 0.2617993874999990922 ) ;
#22296=ORIENTED_EDGE ( 'NONE', *, *, #11897, .T. ) ;
#22330=CYLINDRICAL_SURFACE ( 'NONE', #19201, 0.7874015748031496509 ) ;
#22333=ORIENTED_EDGE ( 'NONE', *, *, #6835, .F. ) ;
#22341=CARTESIAN_POINT ( 'NONE',  ( -2.073220866141732523E-16, 0.07874015748031491790, 1.692913385826771533 ) ) ;
#22359=AXIS2_PLACEMENT_3D ( 'NONE', #20475, #22452, #14123 ) ;
#22370=DIRECTION ( 'NONE',  ( 0.000000000000000000, 0.000000000000000000, -1.000000000000000000 ) ) ;
#22408=FACE_OUTER_BOUND ( 'NONE', #10207, .T. ) ;
#22416=EDGE_CURVE ( 'NONE', #17537, #1638, #894, .T. ) ;
#22422=CYLINDRICAL_SURFACE ( 'NONE', #15508, 0.1181102362204720091 ) ;
#22452=DIRECTION ( 'NONE',  ( -0.000000000000000000, -1.000000000000000000, -0.000000000000000000 ) ) ;
#22462=AXIS2_PLACEMENT_3D ( 'NONE', #7403, #20545, #16173 ) ;
#22482=AXIS2_PLACEMENT_3D ( 'NONE', #11190, #9064, #13313 ) ;
#22485=EDGE_CURVE ( 'NONE', #11993, #19320, #2782, .T. ) ;
#22494=EDGE_CURVE ( 'NONE', #9880, #16039, #11713, .T. ) ;
#22522=ORIENTED_EDGE ( 'NONE', *, *, #11034, .T. ) ;
#22544=AXIS2_PLACEMENT_3D ( 'NONE', #13264, #8883, #177 ) ;
#22562=CARTESIAN_POINT ( 'NONE',  ( 0.000000000000000000, 0.3543307086614172485, 0.000000000000000000 ) ) ;
#22568=CARTESIAN_POINT ( 'NONE',  ( 0.000000000000000000, 0.3937007873309092409, 0.000000000000000000 ) ) ;
#22603=DIRECTION ( 'NONE',  ( 0.000000000000000000, 0.000000000000000000, 1.000000000000000000 ) ) ;
#22605=CYLINDRICAL_SURFACE ( 'NONE', #9668, 1.377952755905512472 ) ;
#22633=CARTESIAN_POINT ( 'NONE',  ( 0.000000000000000000, 0.4724409448818898127, -2.066929133858267598 ) ) ;
#22641=CARTESIAN_POINT ( 'NONE',  ( 1.692913385826771533, 0.07874015748031491790, -0.1181102362204716899 ) ) ;
#22654=DIRECTION ( 'NONE',  ( -0.000000000000000000, -1.000000000000000000, -0.000000000000000000 ) ) ;
#22664=ORIENTED_EDGE ( 'NONE', *, *, #13600, .T. ) ;
#22670=VECTOR ( 'NONE', #16958, 39.37007874015748143 ) ;
#22685=CIRCLE ( 'NONE', #14593, 0.3831516066089791228 ) ;
#22709=AXIS2_PLACEMENT_3D ( 'NONE', #22562, #5326, #20020 ) ;
#22727=CIRCLE ( 'NONE', #11019, 0.1181102362204718703 ) ;
#22747=( LENGTH_UNIT ( ) NAMED_UNIT ( * ) SI_UNIT ( $, .METRE. ) ) ;
#22753=CIRCLE ( 'NONE', #8335, 1.377952755905512472 ) ;
#22763=ORIENTED_EDGE ( 'NONE', *, *, #2812, .T. ) ;
#22777=CARTESIAN_POINT ( 'NONE',  ( 1.197070535079588716, 0.07874015748031495954, 1.315180771300060503 ) ) ;
#22781=ORIENTED_EDGE ( 'NONE', *, *, #13412, .T. ) ;
#22811=EDGE_LOOP ( 'NONE', ( #16492, #3794 ) ) ;
#22832=DIRECTION ( 'NONE',  ( -0.000000000000000000, 1.000000000000000000, -0.000000000000000000 ) ) ;
#22837=VERTEX_POINT ( 'NONE', #10978 ) ;
#22864=AXIS2_PLACEMENT_3D ( 'NONE', #18389, #13747, #22370 ) ;
#22895=DIRECTION ( 'NONE',  ( -0.000000000000000000, -1.000000000000000000, -0.000000000000000000 ) ) ;
#22914=DIRECTION ( 'NONE',  ( 0.000000000000000000, -1.000000000000000000, 0.000000000000000000 ) ) ;
#22918=CIRCLE ( 'NONE', #18837, 0.7874015748031496509 ) ;
#23005=DIRECTION ( 'NONE',  ( -0.000000000000000000, -1.000000000000000000, -0.000000000000000000 ) ) ;
#23018=FACE_BOUND ( 'NONE', #22811, .T. ) ;
#23021=VECTOR ( 'NONE', #27641, 39.37007874015748143 ) ;
#23050=CARTESIAN_POINT ( 'NONE',  ( 0.000000000000000000, 0.1968503937007874127, 0.000000000000000000 ) ) ;
#23088=DIRECTION ( 'NONE',  ( 0.000000000000000000, 0.000000000000000000, -1.000000000000000000 ) ) ;
#23092=DIRECTION ( 'NONE',  ( -0.000000000000000000, -1.000000000000000000, -0.000000000000000000 ) ) ;
#23119=DIRECTION ( 'NONE',  ( 0.000000000000000000, 0.000000000000000000, -1.000000000000000000 ) ) ;
#23135=ORIENTED_EDGE ( 'NONE', *, *, #16858, .T. ) ;
#23172=EDGE_CURVE ( 'NONE', #13858, #372, #9373, .T. ) ;
#23177=CARTESIAN_POINT ( 'NONE',  ( 0.000000000000000000, 0.9055118110236217710, 0.000000000000000000 ) ) ;
#23178=ADVANCED_FACE ( 'NONE', ( #6178 ), #10389, .T. ) ;
#23184=LINE ( 'NONE', #8345, #22670 ) ;
#23212=CARTESIAN_POINT ( 'NONE',  ( 2.531258147843938596E-16, 0.1574803148899641958, 2.066929133858267598 ) ) ;
#23227=ORIENTED_EDGE ( 'NONE', *, *, #3685, .T. ) ;
#23293=CARTESIAN_POINT ( 'NONE',  ( -1.692913385826771533, 0.4724409448818898127, -1.036610629921259805E-16 ) ) ;
#23312=ORIENTED_EDGE ( 'NONE', *, *, #25196, .F. ) ;
#23332=DIRECTION ( 'NONE',  ( 0.000000000000000000, -1.000000000000000000, 0.000000000000000000 ) ) ;
#23351=EDGE_CURVE ( 'NONE', #13627, #7099, #9888, .T. ) ;
#23354=DIRECTION ( 'NONE',  ( -0.000000000000000000, -1.000000000000000000, -0.000000000000000000 ) ) ;
#23373=CARTESIAN_POINT ( 'NONE',  ( 0.000000000000000000, 0.07874015746264864668, 0.000000000000000000 ) ) ;
#23380=CIRCLE ( 'NONE', #11605, 1.377952755905512472 ) ;
#23415=DIRECTION ( 'NONE',  ( -0.000000000000000000, 1.000000000000000000, -0.000000000000000000 ) ) ;
#23418=CONICAL_SURFACE ( 'NONE', #10293, 0.5511811023975373702, 0.7853981633974482790 ) ;
#23421=FILL_AREA_STYLE_COLOUR ( '', #17486 ) ;
#23423=DIRECTION ( 'NONE',  ( 0.000000000000000000, 0.000000000000000000, -1.000000000000000000 ) ) ;
#23438=ORIENTED_EDGE ( 'NONE', *, *, #23172, .T. ) ;
#23484=CARTESIAN_POINT ( 'NONE',  ( 3.874463478174096549E-17, -1.533249767903113305E-16, 0.3163739521363750362 ) ) ;
#23513=CARTESIAN_POINT ( 'NONE',  ( -1.692913385826771533, 0.4724409448818898127, 0.1181102362204718981 ) ) ;
#23519=LINE ( 'NONE', #25484, #7266 ) ;
#23527=ADVANCED_FACE ( 'NONE', ( #4939, #20192 ), #13556, .T. ) ;
#23530=ORIENTED_EDGE ( 'NONE', *, *, #9257, .T. ) ;
#23541=CARTESIAN_POINT ( 'NONE',  ( 0.000000000000000000, 0.3937007873309092409, -2.066929133858267598 ) ) ;
#23542=ORIENTED_EDGE ( 'NONE', *, *, #11034, .F. ) ;
#23558=CARTESIAN_POINT ( 'NONE',  ( 0.000000000000000000, 0.07874015748031495954, -1.692913385826771533 ) ) ;
#23559=DIRECTION ( 'NONE',  ( 0.000000000000000000, 0.000000000000000000, -1.000000000000000000 ) ) ;
#23576=VERTEX_POINT ( 'NONE', #27404 ) ;
#23635=ORIENTED_EDGE ( 'NONE', *, *, #8552, .F. ) ;
#23686=FACE_OUTER_BOUND ( 'NONE', #2181, .T. ) ;
#23692=DIRECTION ( 'NONE',  ( -0.000000000000000000, -1.000000000000000000, -0.000000000000000000 ) ) ;
#23697=CIRCLE ( 'NONE', #27288, 0.2952755905511805778 ) ;
#23716=ORIENTED_EDGE ( 'NONE', *, *, #22494, .T. ) ;
#23721=VECTOR ( 'NONE', #6797, 39.37007874015748143 ) ;
#23748=DIRECTION ( 'NONE',  ( -0.000000000000000000, -1.000000000000000000, -0.000000000000000000 ) ) ;
#23762=DIRECTION ( 'NONE',  ( 0.000000000000000000, 0.000000000000000000, -1.000000000000000000 ) ) ;
#23770=EDGE_LOOP ( 'NONE', ( #15900, #311 ) ) ;
#23796=PRODUCT_DEFINITION_CONTEXT ( 'detailed design', #24776, 'design' ) ;
#23807=VECTOR ( 'NONE', #23692, 39.37007874015748143 ) ;
#23822=( NAMED_UNIT ( * ) PLANE_ANGLE_UNIT ( ) SI_UNIT ( $, .RADIAN. ) ) ;
#23826=ADVANCED_FACE ( 'NONE', ( #2769 ), #22422, .F. ) ;
#23827=AXIS2_PLACEMENT_3D ( 'NONE', #2170, #4437, #10784 ) ;
#23830=ADVANCED_FACE ( 'NONE', ( #15528, #11679 ), #20301, .F. ) ;
#23836=CARTESIAN_POINT ( 'NONE',  ( 1.446433227339387294E-17, 0.07874015748031491790, -1.574803149606299524 ) ) ;
#23885=LINE ( 'NONE', #18930, #1635 ) ;
#23908=DIRECTION ( 'NONE',  ( 0.000000000000000000, 0.000000000000000000, -1.000000000000000000 ) ) ;
#23913=VERTEX_POINT ( 'NONE', #24393 ) ;
#23952=EDGE_CURVE ( 'NONE', #17381, #14467, #22727, .T. ) ;
#23955=CARTESIAN_POINT ( 'NONE',  ( 0.000000000000000000, 0.4724409448818896462, 0.000000000000000000 ) ) ;
#23984=AXIS2_PLACEMENT_3D ( 'NONE', #21714, #13220, #10 ) ;
#24017=CYLINDRICAL_SURFACE ( 'NONE', #3036, 2.066929133858267598 ) ;
#24019=EDGE_CURVE ( 'NONE', #10268, #12707, #1082, .T. ) ;
#24034=ORIENTED_EDGE ( 'NONE', *, *, #6709, .F. ) ;
#24039=FACE_BOUND ( 'NONE', #14731, .T. ) ;
#24043=ORIENTED_EDGE ( 'NONE', *, *, #24503, .T. ) ;
#24080=DIRECTION ( 'NONE',  ( -0.000000000000000000, -1.000000000000000000, -0.000000000000000000 ) ) ;
#24117=EDGE_LOOP ( 'NONE', ( #14109, #24648, #13102, #3070 ) ) ;
#24147=DIRECTION ( 'NONE',  ( 0.000000000000000000, 0.000000000000000000, -1.000000000000000000 ) ) ;
#24150=EDGE_LOOP ( 'NONE', ( #249, #23438, #14698, #8446 ) ) ;
#24155=CARTESIAN_POINT ( 'NONE',  ( 1.687505431895960050E-16, 0.1968503937007875237, 1.377952755905512472 ) ) ;
#24173=EDGE_CURVE ( 'NONE', #6614, #10848, #16383, .T. ) ;
#24215=VERTEX_POINT ( 'NONE', #15577 ) ;
#24232=AXIS2_PLACEMENT_3D ( 'NONE', #9455, #20351, #26989 ) ;
#24289=ADVANCED_FACE ( 'NONE', ( #15447, #17670, #6405, #10623, #19249, #26161, #8513, #17133, #17547, #24039 ), #4676, .T. ) ;
#24294=DIRECTION ( 'NONE',  ( 0.000000000000000000, 0.000000000000000000, 1.000000000000000000 ) ) ;
#24314=CARTESIAN_POINT ( 'NONE',  ( 1.197070535079588716, 0.07874015748031491790, -1.078960298859116707 ) ) ;
#24340=DIRECTION ( 'NONE',  ( -0.000000000000000000, -1.000000000000000000, -0.000000000000000000 ) ) ;
#24374=EDGE_LOOP ( 'NONE', ( #19237, #17842, #14876, #3736 ) ) ;
#24393=CARTESIAN_POINT ( 'NONE',  ( 1.197070535079588716, 0.07874015748031491790, 1.078960298859116707 ) ) ;
#24401=ORIENTED_EDGE ( 'NONE', *, *, #15982, .T. ) ;
#24409=ORIENTED_EDGE ( 'NONE', *, *, #17691, .F. ) ;
#24413=AXIS2_PLACEMENT_3D ( 'NONE', #1012, #26560, #5091 ) ;
#24434=CYLINDRICAL_SURFACE ( 'NONE', #21454, 0.1181102362204718703 ) ;
#24437=CARTESIAN_POINT ( 'NONE',  ( -1.197070535079588716, 0.07874015748031495954, -1.315180771300060503 ) ) ;
#24479=EDGE_CURVE ( 'NONE', #7932, #8591, #9196, .T. ) ;
#24481=EDGE_LOOP ( 'NONE', ( #17205, #12263 ) ) ;
#24494=AXIS2_PLACEMENT_3D ( 'NONE', #22341, #11601, #3245 ) ;
#24501=VECTOR ( 'NONE', #24668, 39.37007874015748143 ) ;
#24503=EDGE_CURVE ( 'NONE', #7615, #15934, #20490, .T. ) ;
#24515=VERTEX_POINT ( 'NONE', #12616 ) ;
#24527=CARTESIAN_POINT ( 'NONE',  ( -1.692913385826771533, 0.07874015748031495954, -1.036610629921259805E-16 ) ) ;
#24537=EDGE_LOOP ( 'NONE', ( #15027, #21310 ) ) ;
#24569=CIRCLE ( 'NONE', #17806, 1.377952755905512472 ) ;
#24631=AXIS2_PLACEMENT_3D ( 'NONE', #7681, #17956, #26731 ) ;
#24633=LINE ( 'NONE', #12353, #7643 ) ;
#24637=CARTESIAN_POINT ( 'NONE',  ( 0.000000000000000000, 0.9055118110236221041, 0.000000000000000000 ) ) ;
#24648=ORIENTED_EDGE ( 'NONE', *, *, #3494, .T. ) ;
#24650=CARTESIAN_POINT ( 'NONE',  ( 0.000000000000000000, 0.4724409448818898127, -1.692913385826771533 ) ) ;
#24653=EDGE_LOOP ( 'NONE', ( #5783, #12767 ) ) ;
#24668=DIRECTION ( 'NONE',  ( -0.000000000000000000, -1.000000000000000000, -0.000000000000000000 ) ) ;
#24672=EDGE_CURVE ( 'NONE', #15934, #7615, #18204, .T. ) ;
#24693=DIRECTION ( 'NONE',  ( -0.000000000000000000, 1.000000000000000000, -0.000000000000000000 ) ) ;
#24694=DIRECTION ( 'NONE',  ( -0.000000000000000000, 1.000000000000000000, -0.000000000000000000 ) ) ;
#24721=DIRECTION ( 'NONE',  ( -0.000000000000000000, -1.000000000000000000, -0.000000000000000000 ) ) ;
#24763=DIRECTION ( 'NONE',  ( 0.000000000000000000, -1.000000000000000000, 0.000000000000000000 ) ) ;
#24776=APPLICATION_CONTEXT ( 'automotive_design' ) ;
#24780=ADVANCED_FACE ( 'NONE', ( #4228 ), #12562, .T. ) ;
#24792=DIRECTION ( 'NONE',  ( 0.000000000000000000, 0.000000000000000000, -1.000000000000000000 ) ) ;
#24824=DIRECTION ( 'NONE',  ( 0.000000000000000000, 0.000000000000000000, -1.000000000000000000 ) ) ;
#24844=ADVANCED_FACE ( 'NONE', ( #25697 ), #1820, .F. ) ;
#24851=UNCERTAINTY_MEASURE_WITH_UNIT (LENGTH_MEASURE( 1.000000000000000082E-05 ), #26069, 'distance_accuracy_value', 'NONE') ;
#24878=CARTESIAN_POINT ( 'NONE',  ( 0.000000000000000000, 0.07874015748662489822, 0.000000000000000000 ) ) ;
#24879=EDGE_LOOP ( 'NONE', ( #10167, #14231, #10972, #1432 ) ) ;
#24901=ORIENTED_EDGE ( 'NONE', *, *, #11136, .T. ) ;
#24908=FACE_OUTER_BOUND ( 'NONE', #2961, .T. ) ;
#24917=ADVANCED_FACE ( 'NONE', ( #10998, #22139 ), #7166, .T. ) ;
#24952=LINE ( 'NONE', #16069, #13434 ) ;
#24988=ORIENTED_EDGE ( 'NONE', *, *, #27793, .F. ) ;
#25005=CARTESIAN_POINT ( 'NONE',  ( 0.000000000000000000, 0.1968503937007875237, 0.000000000000000000 ) ) ;
#25041=VECTOR ( 'NONE', #7501, 39.37007874015748143 ) ;
#25052=CARTESIAN_POINT ( 'NONE',  ( 0.000000000000000000, 0.07874015748031495954, 0.000000000000000000 ) ) ;
#25055=AXIS2_PLACEMENT_3D ( 'NONE', #4838, #16421, #9341 ) ;
#25057=LINE ( 'NONE', #19224, #13768 ) ;
#25082=DIRECTION ( 'NONE',  ( 0.000000000000000000, 0.000000000000000000, -1.000000000000000000 ) ) ;
#25121=FACE_BOUND ( 'NONE', #12736, .T. ) ;
#25145=VERTEX_POINT ( 'NONE', #8426 ) ;
#25146=VECTOR ( 'NONE', #11226, 39.37007874015748143 ) ;
#25159=ORIENTED_EDGE ( 'NONE', *, *, #11979, .T. ) ;
#25175=AXIS2_PLACEMENT_3D ( 'NONE', #8009, #23415, #10110 ) ;
#25196=EDGE_CURVE ( 'NONE', #27656, #16023, #17046, .T. ) ;
#25200=ORIENTED_EDGE ( 'NONE', *, *, #16048, .F. ) ;
#25202=AXIS2_PLACEMENT_3D ( 'NONE', #11583, #26688, #7349 ) ;
#25227=ORIENTED_EDGE ( 'NONE', *, *, #19993, .F. ) ;
#25230=EDGE_CURVE ( 'NONE', #152, #4045, #18244, .T. ) ;
#25263=FACE_BOUND ( 'NONE', #911, .T. ) ;
#25264=ORIENTED_EDGE ( 'NONE', *, *, #21289, .F. ) ;
#25306=DIRECTION ( 'NONE',  ( 0.000000000000000000, 0.000000000000000000, -1.000000000000000000 ) ) ;
#25308=VERTEX_POINT ( 'NONE', #26070 ) ;
#25316=ORIENTED_EDGE ( 'NONE', *, *, #27857, .T. ) ;
#25330=CARTESIAN_POINT ( 'NONE',  ( 0.000000000000000000, 0.3543307086614172485, 0.000000000000000000 ) ) ;
#25337=DIRECTION ( 'NONE',  ( -0.000000000000000000, 1.000000000000000000, 0.000000000000000000 ) ) ;
#25345=ORIENTED_EDGE ( 'NONE', *, *, #24479, .T. ) ;
#25362=VECTOR ( 'NONE', #16103, 39.37007874015748143 ) ;
#25371=AXIS2_PLACEMENT_3D ( 'NONE', #14674, #264, #23559 ) ;
#25393=VERTEX_POINT ( 'NONE', #9097 ) ;
#25405=ORIENTED_EDGE ( 'NONE', *, *, #5192, .T. ) ;
#25419=CARTESIAN_POINT ( 'NONE',  ( 1.197070535079588716, 0.07874015748031491790, -1.197070535079588716 ) ) ;
#25461=ORIENTED_EDGE ( 'NONE', *, *, #25627, .T. ) ;
#25477=EDGE_CURVE ( 'NONE', #8591, #7932, #23697, .T. ) ;
#25478=CIRCLE ( 'NONE', #18219, 0.4921259842519685179 ) ;
#25484=CARTESIAN_POINT ( 'NONE',  ( 0.000000000000000000, 0.9055118110236221041, -0.3937007874015748254 ) ) ;
#25487=FACE_BOUND ( 'NONE', #21300, .T. ) ;
#25503=ORIENTED_EDGE ( 'NONE', *, *, #9101, .T. ) ;
#25509=VERTEX_POINT ( 'NONE', #27010 ) ;
#25521=FACE_BOUND ( 'NONE', #24481, .T. ) ;
#25620=CARTESIAN_POINT ( 'NONE',  ( 3.616083068348477634E-17, 0.07874015748662489822, 0.2952755905511805778 ) ) ;
#25623=ORIENTED_EDGE ( 'NONE', *, *, #21093, .F. ) ;
#25625=DIRECTION ( 'NONE',  ( 0.000000000000000000, 0.000000000000000000, 1.000000000000000000 ) ) ;
#25627=EDGE_CURVE ( 'NONE', #23576, #11604, #13006, .T. ) ;
#25642=CIRCLE ( 'NONE', #13443, 0.7874015748208159637 ) ;
#25697=FACE_OUTER_BOUND ( 'NONE', #9530, .T. ) ;
#25728=DIRECTION ( 'NONE',  ( 0.000000000000000000, -1.000000000000000000, 0.000000000000000000 ) ) ;
#25735=CARTESIAN_POINT ( 'NONE',  ( 0.000000000000000000, 0.07874015748031495954, -1.692913385826771533 ) ) ;
#25760=CARTESIAN_POINT ( 'NONE',  ( 1.692913385826771533, 0.4724409448818898127, 3.109831496062992451E-16 ) ) ;
#25773=ORIENTED_EDGE ( 'NONE', *, *, #33, .T. ) ;
#25797=PLANE ( 'NONE',  #20732 ) ;
#25815=ORIENTED_EDGE ( 'NONE', *, *, #6709, .T. ) ;
#25827=DIRECTION ( 'NONE',  ( 0.000000000000000000, 0.000000000000000000, -1.000000000000000000 ) ) ;
#25848=ORIENTED_EDGE ( 'NONE', *, *, #21441, .T. ) ;
#25852=EDGE_LOOP ( 'NONE', ( #27322, #17864 ) ) ;
#25874=DIRECTION ( 'NONE',  ( 0.000000000000000000, 0.000000000000000000, 1.000000000000000000 ) ) ;
#25923=ORIENTED_EDGE ( 'NONE', *, *, #3120, .F. ) ;
#25934=LINE ( 'NONE', #15078, #23807 ) ;
#25940=AXIS2_PLACEMENT_3D ( 'NONE', #17533, #4801, #6389 ) ;
#25976=EDGE_CURVE ( 'NONE', #18301, #26351, #25057, .T. ) ;
#26021=ORIENTED_EDGE ( 'NONE', *, *, #4475, .F. ) ;
#26062=DIRECTION ( 'NONE',  ( 0.000000000000000000, 0.000000000000000000, 1.000000000000000000 ) ) ;
#26069=( CONVERSION_BASED_UNIT ( 'INCH', #26201 ) LENGTH_UNIT ( ) NAMED_UNIT ( #18919 ) ) ;
#26070=CARTESIAN_POINT ( 'NONE',  ( 4.821444091131312140E-17, 0.03937007874015747977, 0.3937007874015748254 ) ) ;
#26072=CIRCLE ( 'NONE', #13885, 0.3937007874015748254 ) ;
#26082=CYLINDRICAL_SURFACE ( 'NONE', #23984, 0.1181102362204720091 ) ;
#26114=CIRCLE ( 'NONE', #4459, 0.2952755905511805223 ) ;
#26124=EDGE_CURVE ( 'NONE', #14972, #7615, #26404, .T. ) ;
#26133=DIRECTION ( 'NONE',  ( 0.000000000000000000, 0.000000000000000000, -1.000000000000000000 ) ) ;
#26161=FACE_BOUND ( 'NONE', #3459, .T. ) ;
#26166=DIRECTION ( 'NONE',  ( -0.000000000000000000, -1.000000000000000000, -0.000000000000000000 ) ) ;
#26201=LENGTH_MEASURE_WITH_UNIT ( LENGTH_MEASURE( 0.02539999999999999897 ), #2328 ) ;
#26212=EDGE_CURVE ( 'NONE', #7459, #247, #13690, .T. ) ;
#26268=VECTOR ( 'NONE', #18901, 39.37007874015748143 ) ;
#26276=EDGE_CURVE ( 'NONE', #23913, #19458, #2514, .T. ) ;
#26284=LINE ( 'NONE', #15571, #5636 ) ;
#26290=VERTEX_POINT ( 'NONE', #26976 ) ;
#26291=CARTESIAN_POINT ( 'NONE',  ( 0.000000000000000000, 0.1968503937007874127, 0.000000000000000000 ) ) ;
#26316=DIRECTION ( 'NONE',  ( 0.000000000000000000, 0.000000000000000000, 1.000000000000000000 ) ) ;
#26317=FACE_OUTER_BOUND ( 'NONE', #1250, .T. ) ;
#26334=FACE_OUTER_BOUND ( 'NONE', #24117, .T. ) ;
#26337=LINE ( 'NONE', #15756, #25146 ) ;
#26346=AXIS2_PLACEMENT_3D ( 'NONE', #4759, #9000, #13654 ) ;
#26351=VERTEX_POINT ( 'NONE', #7128 ) ;
#26374=DIRECTION ( 'NONE',  ( 0.000000000000000000, 0.000000000000000000, -1.000000000000000000 ) ) ;
#26392=DIRECTION ( 'NONE',  ( 0.000000000000000000, 0.000000000000000000, -1.000000000000000000 ) ) ;
#26404=LINE ( 'NONE', #17521, #23721 ) ;
#26412=FACE_BOUND ( 'NONE', #16316, .T. ) ;
#26419=ORIENTED_EDGE ( 'NONE', *, *, #9101, .F. ) ;
#26464=AXIS2_PLACEMENT_3D ( 'NONE', #20088, #16409, #12311 ) ;
#26550=ADVANCED_FACE ( 'NONE', ( #5232 ), #22330, .T. ) ;
#26560=DIRECTION ( 'NONE',  ( -0.000000000000000000, 1.000000000000000000, -0.000000000000000000 ) ) ;
#26563=VECTOR ( 'NONE', #26166, 39.37007874015748143 ) ;
#26579=AXIS2_PLACEMENT_3D ( 'NONE', #7677, #14180, #12708 ) ;
#26593=ADVANCED_FACE ( 'NONE', ( #17924 ), #17668, .T. ) ;
#26607=DIRECTION ( 'NONE',  ( 0.000000000000000000, -1.000000000000000000, 0.000000000000000000 ) ) ;
#26650=LINE ( 'NONE', #1107, #24501 ) ;
#26664=ORIENTED_EDGE ( 'NONE', *, *, #27822, .T. ) ;
#26683=EDGE_LOOP ( 'NONE', ( #22086, #27136, #9389, #18109 ) ) ;
#26686=CARTESIAN_POINT ( 'NONE',  ( 1.692913385826771533, 0.07874015748031491790, 3.109831496062992451E-16 ) ) ;
#26688=DIRECTION ( 'NONE',  ( -0.000000000000000000, -1.000000000000000000, -0.000000000000000000 ) ) ;
#26696=AXIS2_PLACEMENT_3D ( 'NONE', #14566, #18617, #14272 ) ;
#26697=DIRECTION ( 'NONE',  ( 0.000000000000000000, -1.000000000000000000, 0.000000000000000000 ) ) ;
#26698=LINE ( 'NONE', #24437, #7590 ) ;
#26731=DIRECTION ( 'NONE',  ( 0.000000000000000000, 0.000000000000000000, 1.000000000000000000 ) ) ;
#26748=DIRECTION ( 'NONE',  ( -0.000000000000000000, -1.000000000000000000, -0.000000000000000000 ) ) ;
#26755=DIRECTION ( 'NONE',  ( 0.000000000000000000, 0.000000000000000000, 1.000000000000000000 ) ) ;
#26782=ORIENTED_EDGE ( 'NONE', *, *, #20571, .T. ) ;
#26834=ORIENTED_EDGE ( 'NONE', *, *, #16048, .T. ) ;
#26840=CYLINDRICAL_SURFACE ( 'NONE', #10580, 0.3937007874015748254 ) ;
#26851=AXIS2_PLACEMENT_3D ( 'NONE', #25330, #12751, #14323 ) ;
#26852=EDGE_CURVE ( 'NONE', #13490, #25509, #23885, .T. ) ;
#26856=CARTESIAN_POINT ( 'NONE',  ( -1.692913385826771533, 0.4724409448818898127, -0.1181102362204721062 ) ) ;
#26953=DIRECTION ( 'NONE',  ( 0.000000000000000000, -1.000000000000000000, 0.000000000000000000 ) ) ;
#26976=CARTESIAN_POINT ( 'NONE',  ( 0.000000000000000000, -1.707404996040164512E-16, -0.3937007874015748254 ) ) ;
#26989=DIRECTION ( 'NONE',  ( 0.000000000000000000, 0.000000000000000000, -1.000000000000000000 ) ) ;
#26993=ADVANCED_FACE ( 'NONE', ( #13128 ), #837, .F. ) ;
#27008=CARTESIAN_POINT ( 'NONE',  ( -1.197070535079588716, 0.07874015748031491790, 1.315180771300060503 ) ) ;
#27010=CARTESIAN_POINT ( 'NONE',  ( 0.000000000000000000, 0.4724409448818898127, -0.4921259842519685179 ) ) ;
#27037=EDGE_LOOP ( 'NONE', ( #9490, #25200, #12630, #22763 ) ) ;
#27049=LINE ( 'NONE', #17970, #22231 ) ;
#27050=AXIS2_PLACEMENT_3D ( 'NONE', #15328, #17147, #25625 ) ;
#27055=ADVANCED_FACE ( 'NONE', ( #13271 ), #6784, .F. ) ;
#27061=ORIENTED_EDGE ( 'NONE', *, *, #10592, .F. ) ;
#27064=ORIENTED_EDGE ( 'NONE', *, *, #13600, .F. ) ;
#27071=ORIENTED_EDGE ( 'NONE', *, *, #114, .T. ) ;
#27080=CARTESIAN_POINT ( 'NONE',  ( 9.642888182478974314E-17, 0.07874015746264864668, 0.7874015748208159637 ) ) ;
#27115=FACE_OUTER_BOUND ( 'NONE', #15512, .T. ) ;
#27133=DIRECTION ( 'NONE',  ( 0.000000000000000000, 0.000000000000000000, 1.000000000000000000 ) ) ;
#27136=ORIENTED_EDGE ( 'NONE', *, *, #24479, .F. ) ;
#27142=CARTESIAN_POINT ( 'NONE',  ( 0.000000000000000000, 0.1968503937007875237, -0.7874015748208159637 ) ) ;
#27144=EDGE_LOOP ( 'NONE', ( #25815, #23227 ) ) ;
#27145=ORIENTED_EDGE ( 'NONE', *, *, #19328, .F. ) ;
#27151=EDGE_CURVE ( 'NONE', #27656, #13490, #18783, .T. ) ;
#27167=DIRECTION ( 'NONE',  ( 8.659560554583420347E-17, -0.7071067818211396183, 0.7071067805519553051 ) ) ;
#27168=VERTEX_POINT ( 'NONE', #8178 ) ;
#27179=EDGE_LOOP ( 'NONE', ( #27071, #1636, #8822, #23635 ) ) ;
#27210=DIRECTION ( 'NONE',  ( 0.000000000000000000, 0.000000000000000000, -1.000000000000000000 ) ) ;
#27211=DIRECTION ( 'NONE',  ( 0.000000000000000000, -1.000000000000000000, 0.000000000000000000 ) ) ;
#27288=AXIS2_PLACEMENT_3D ( 'NONE', #24878, #22914, #25306 ) ;
#27299=CONICAL_SURFACE ( 'NONE', #21877, 0.2952755905511805778, 0.2617993875000016457 ) ;
#27317=CARTESIAN_POINT ( 'NONE',  ( 1.197070535079588716, 0.07874015748031495954, -1.078960298859116707 ) ) ;
#27319=CARTESIAN_POINT ( 'NONE',  ( 1.197070535079588716, 0.4724409448818898127, 1.315180771300060503 ) ) ;
#27322=ORIENTED_EDGE ( 'NONE', *, *, #19106, .F. ) ;
#27329=VERTEX_POINT ( 'NONE', #21828 ) ;
#27331=AXIS2_PLACEMENT_3D ( 'NONE', #26291, #6953, #15575 ) ;
#27359=CARTESIAN_POINT ( 'NONE',  ( 0.000000000000000000, 0.1968503937007874127, 0.000000000000000000 ) ) ;
#27364=CARTESIAN_POINT ( 'NONE',  ( 6.026805113914139867E-17, 0.9055118110236221041, 0.4921259842519685179 ) ) ;
#27381=EDGE_CURVE ( 'NONE', #12564, #17190, #19709, .T. ) ;
#27397=CIRCLE ( 'NONE', #2124, 0.3937007874015748254 ) ;
#27400=LINE ( 'NONE', #11851, #26268 ) ;
#27404=CARTESIAN_POINT ( 'NONE',  ( -1.928577543407793639E-16, 0.4724409448818898127, 1.811023622047243542 ) ) ;
#27408=DIRECTION ( 'NONE',  ( 0.000000000000000000, -1.000000000000000000, 0.000000000000000000 ) ) ;
#27410=ORIENTED_EDGE ( 'NONE', *, *, #5649, .T. ) ;
#27420=ORIENTED_EDGE ( 'NONE', *, *, #10264, .T. ) ;
#27424=CARTESIAN_POINT ( 'NONE',  ( -1.197070535079588716, 0.4724409448818898127, 1.315180771300060503 ) ) ;
#27435=CIRCLE ( 'NONE', #20205, 0.5511811023975373702 ) ;
#27442=DIRECTION ( 'NONE',  ( 0.000000000000000000, -1.000000000000000000, 0.000000000000000000 ) ) ;
#27465=EDGE_CURVE ( 'NONE', #12080, #12707, #7827, .T. ) ;
#27474=CIRCLE ( 'NONE', #25202, 0.1181102362204720091 ) ;
#27504=DIRECTION ( 'NONE',  ( 0.000000000000000000, -1.000000000000000000, 0.000000000000000000 ) ) ;
#27506=EDGE_CURVE ( 'NONE', #12497, #26290, #4366, .T. ) ;
#27510=CARTESIAN_POINT ( 'NONE',  ( 0.000000000000000000, 0.07874015748031508444, 0.000000000000000000 ) ) ;
#27516=ORIENTED_EDGE ( 'NONE', *, *, #14872, .T. ) ;
#27543=CARTESIAN_POINT ( 'NONE',  ( 2.483043706889356121E-16, 0.07874015748031495954, -1.988188976307287970 ) ) ;
#27589=CARTESIAN_POINT ( 'NONE',  ( 0.000000000000000000, 0.9055118110236217710, 0.000000000000000000 ) ) ;
#27592=EDGE_CURVE ( 'NONE', #3555, #17381, #27850, .T. ) ;
#27601=LINE ( 'NONE', #8244, #3379 ) ;
#27609=EDGE_LOOP ( 'NONE', ( #629, #15705, #7725, #22333 ) ) ;
#27611=FACE_OUTER_BOUND ( 'NONE', #24537, .T. ) ;
#27641=DIRECTION ( 'NONE',  ( -0.000000000000000000, -1.000000000000000000, -0.000000000000000000 ) ) ;
#27656=VERTEX_POINT ( 'NONE', #20811 ) ;
#27668=EDGE_CURVE ( 'NONE', #6614, #25145, #15221, .T. ) ;
#27672=CARTESIAN_POINT ( 'NONE',  ( 0.000000000000000000, 0.5905511811023621549, 0.000000000000000000 ) ) ;
#27674=ORIENTED_EDGE ( 'NONE', *, *, #10642, .F. ) ;
#27675=AXIS2_PLACEMENT_3D ( 'NONE', #4079, #3937, #10560 ) ;
#27679=DIRECTION ( 'NONE',  ( 0.000000000000000000, 0.000000000000000000, -1.000000000000000000 ) ) ;
#27793=EDGE_CURVE ( 'NONE', #16039, #9880, #16549, .T. ) ;
#27822=EDGE_CURVE ( 'NONE', #11993, #14551, #27866, .T. ) ;
#27825=VECTOR ( 'NONE', #22654, 39.37007874015748143 ) ;
#27833=FACE_OUTER_BOUND ( 'NONE', #12652, .T. ) ;
#27850=LINE ( 'NONE', #27317, #6633 ) ;
#27857=EDGE_CURVE ( 'NONE', #26290, #12497, #27397, .T. ) ;
#27862=DIRECTION ( 'NONE',  ( -0.000000000000000000, 1.000000000000000000, -0.000000000000000000 ) ) ;
#27866=CIRCLE ( 'NONE', #24232, 0.5511811023975373702 ) ;
#27867=AXIS2_PLACEMENT_3D ( 'NONE', #20583, #18728, #10246 ) ;
ENDSEC;
END-ISO-10303-21;
